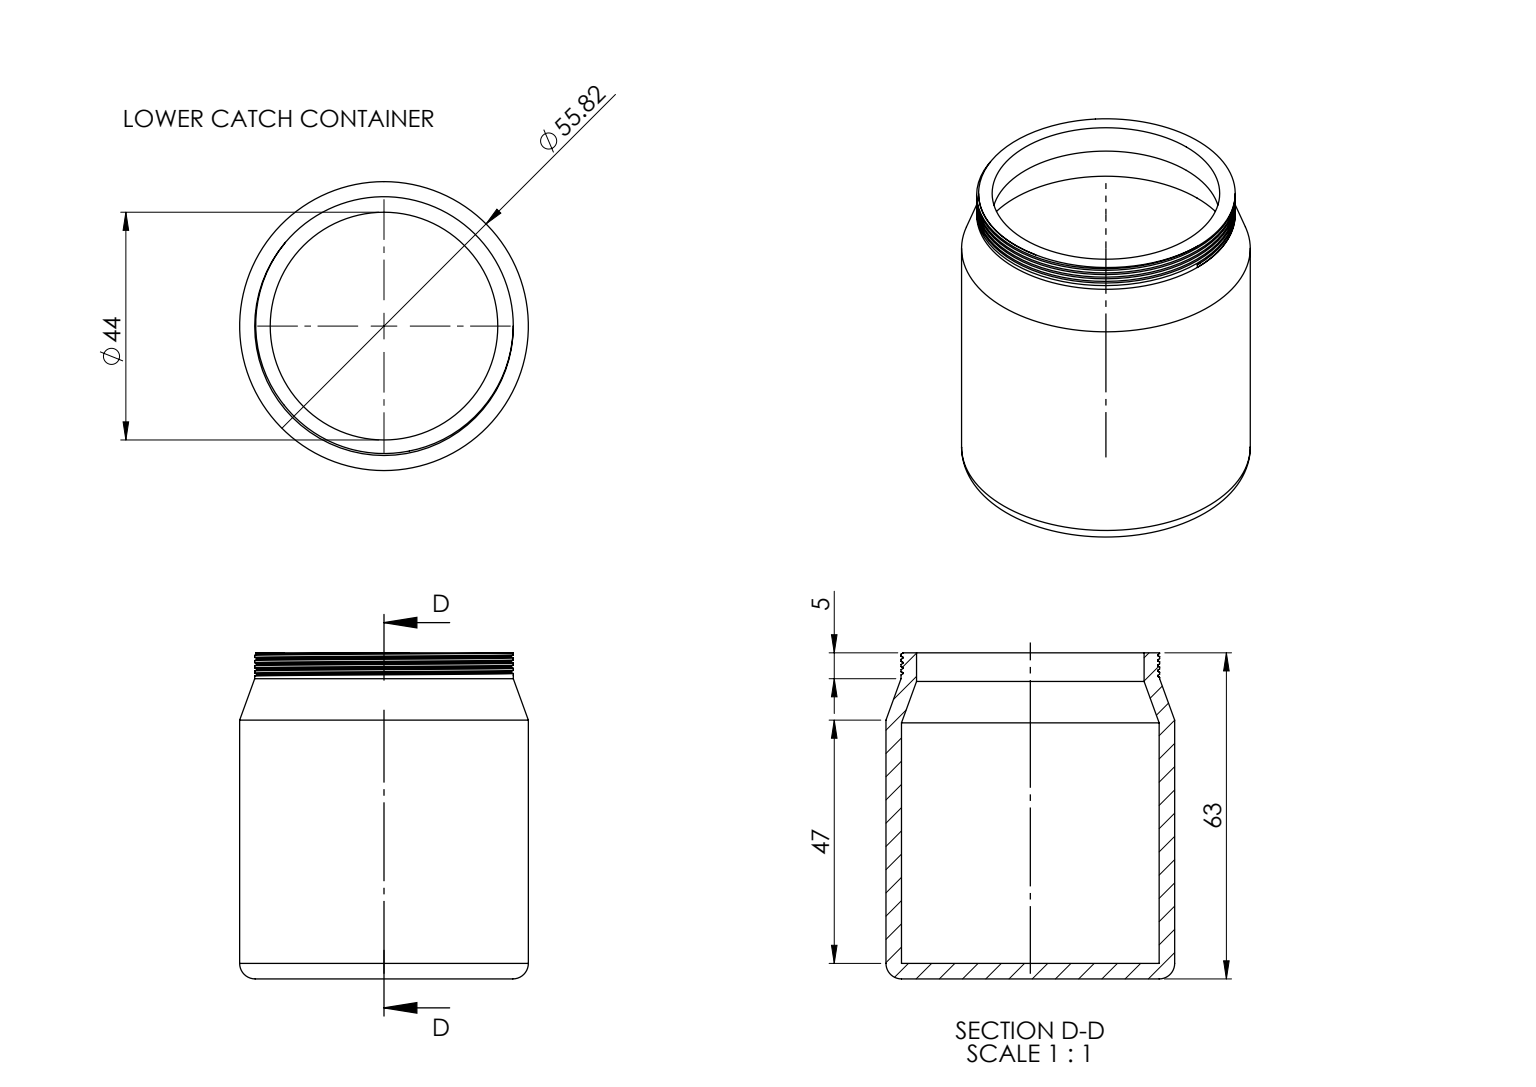
ISO-10303-21;
HEADER;
FILE_DESCRIPTION (('STEP AP214'),
    '1' );
FILE_NAME ('Lower Catch Container.step',
    '2026-10-04T07:23:31',
    ( '' ),
    ( '' ),
    'SwSTEP 2.0',
    'SolidWorks 2026',
    '' );
FILE_SCHEMA (( 'AUTOMOTIVE_DESIGN' ));
ENDSEC;

DATA;
#7=CARTESIAN_POINT ( 'NONE',  ( -10.19839929293505776, 0.5312499990440845421, -24.62111388750000174 ) ) ;
#10=CARTESIAN_POINT ( 'NONE',  ( 1.530808498934191521E-15, 3.250000000000000444, -25.00000000000000000 ) ) ;
#15=CARTESIAN_POINT ( 'NONE',  ( 24.62111388749999463, 5.156249999044083765, 10.19839929293507730 ) ) ;
#16=FACE_OUTER_BOUND ( 'NONE', #4981, .T. ) ;
#25=DIRECTION ( 'NONE',  ( 0.000000000000000000, 0.000000000000000000, -1.000000000000000000 ) ) ;
#39=VERTEX_POINT ( 'NONE', #260 ) ;
#48=TOROIDAL_SURFACE ( 'NONE', #9050, 24.91176187412963117, 3.000000000000000000 ) ;
#50=EDGE_CURVE ( 'NONE', #1424, #5838, #3619, .T. ) ;
#51=CARTESIAN_POINT ( 'NONE',  ( -10.19839929293507552, 1.081249999044084475, 24.62111388749999463 ) ) ;
#52=CARTESIAN_POINT ( 'NONE',  ( -10.19839929293505776, 1.706249999044084698, -24.62111388750000174 ) ) ;
#57=VERTEX_POINT ( 'NONE', #5944 ) ;
#59=FILL_AREA_STYLE_COLOUR ( '', #6484 ) ;
#69=VERTEX_POINT ( 'NONE', #5118 ) ;
#70=UNCERTAINTY_MEASURE_WITH_UNIT (LENGTH_MEASURE( 1.000000000000000082E-05 ), #3920, 'distance_accuracy_value', 'NONE');
#72=CARTESIAN_POINT ( 'NONE',  ( -10.19839929293507552, 0.9062499990440844311, 24.62111388749999463 ) ) ;
#79=CARTESIAN_POINT ( 'NONE',  ( 0.000000000000000000, 5.000000000000000000, 0.000000000000000000 ) ) ;
#80=CARTESIAN_POINT ( 'NONE',  ( -17.67766952966369232, 0.6250000000000000000, 17.67766952966368876 ) ) ;
#81=CARTESIAN_POINT ( 'NONE',  ( -25.00000000000000000, 3.112499998088169129, -3.061616997868383043E-15 ) ) ;
#90=FACE_OUTER_BOUND ( 'NONE', #9620, .T. ) ;
#98=CARTESIAN_POINT ( 'NONE',  ( 24.62111388750000174, 0.4562499990440845310, -10.19839929293505776 ) ) ;
#107=CARTESIAN_POINT ( 'NONE',  ( -4.522825247065398226E-15, 3.143749999044084475, 24.62111388750000174 ) ) ;
#116=CARTESIAN_POINT ( 'NONE',  ( -25.00000000000000000, 2.112499998088169129, -3.061616997868383043E-15 ) ) ;
#118=CARTESIAN_POINT ( 'NONE',  ( 17.67766952966368521, 2.875000000000000000, 17.67766952966369232 ) ) ;
#125=CARTESIAN_POINT ( 'NONE',  ( -10.19839929293507552, 5.081249999044084475, 24.62111388749999463 ) ) ;
#135=CARTESIAN_POINT ( 'NONE',  ( -25.00000000000000000, 0.4375000000000000000, -10.35533905932738108 ) ) ;
#137=EDGE_LOOP ( 'NONE', ( #3283, #4277, #3194, #1557 ) ) ;
#158=CARTESIAN_POINT ( 'NONE',  ( -24.62111388750000174, 4.831249999044084475, -10.19839929293506131 ) ) ;
#164=CARTESIAN_POINT ( 'NONE',  ( -10.19839929293505776, 0.7062499990440844755, -24.62111388750000174 ) ) ;
#166=CARTESIAN_POINT ( 'NONE',  ( -25.00000000000000000, 1.049999998088169129, -10.35533905932738108 ) ) ;
#172=CARTESIAN_POINT ( 'NONE',  ( 10.19839929293505953, 0.4062499990440845421, -24.62111388750000174 ) ) ;
#175=CARTESIAN_POINT ( 'NONE',  ( -25.00000000000001421, 3.562500000000000444, 10.35533905932737397 ) ) ;
#183=LINE ( 'NONE', #1845, #502 ) ;
#184=CARTESIAN_POINT ( 'NONE',  ( 24.62111388749999463, 4.331249999044085364, 10.19839929293507730 ) ) ;
#193=DIRECTION ( 'NONE',  ( 0.000000000000000000, 0.000000000000000000, -1.000000000000000000 ) ) ;
#195=CARTESIAN_POINT ( 'NONE',  ( -10.35533905932737575, 1.312500000000000444, -25.00000000000000000 ) ) ;
#197=CARTESIAN_POINT ( 'NONE',  ( -17.67766952966369232, 3.237499998088169573, 17.67766952966368876 ) ) ;
#204=EDGE_CURVE ( 'NONE', #10138, #4764, #1958, .T. ) ;
#218=CARTESIAN_POINT ( 'NONE',  ( 17.40975659021752975, 4.518749999044084475, -17.40975659021752975 ) ) ;
#228=CARTESIAN_POINT ( 'NONE',  ( -24.62111388750000174, 1.831249999044084475, -10.19839929293506131 ) ) ;
#237=CARTESIAN_POINT ( 'NONE',  ( -24.62111388750000174, 0.6562499990440845421, -10.19839929293506131 ) ) ;
#240=AXIS2_PLACEMENT_3D ( 'NONE', #1921, #5301, #7838 ) ;
#245=CARTESIAN_POINT ( 'NONE',  ( 17.40975659021752975, 3.518749999044084920, -17.40975659021752975 ) ) ;
#254=CARTESIAN_POINT ( 'NONE',  ( -25.00000000000000000, 1.437500000000000000, -10.35533905932738108 ) ) ;
#256=EDGE_CURVE ( 'NONE', #8849, #3847, #4015, .T. ) ;
#260=CARTESIAN_POINT ( 'NONE',  ( 1.530808498934191521E-15, 0.8624999980881691286, -25.00000000000000000 ) ) ;
#262=FACE_OUTER_BOUND ( 'NONE', #1288, .T. ) ;
#270=EDGE_LOOP ( 'NONE', ( #6260, #9302, #1877, #7015, #4822 ) ) ;
#273=CARTESIAN_POINT ( 'NONE',  ( 24.99999999999999289, 2.937500000000000000, 10.35533905932739529 ) ) ;
#274=CARTESIAN_POINT ( 'NONE',  ( 10.35533905932738286, 1.424999998088169129, 24.99999999999999645 ) ) ;
#275=CARTESIAN_POINT ( 'NONE',  ( 17.40975659021752975, 3.518749999044084920, -17.40975659021752975 ) ) ;
#282=CARTESIAN_POINT ( 'NONE',  ( 10.19839929293506486, 5.206249999044084475, 24.62111388749999819 ) ) ;
#286=ORIENTED_EDGE ( 'NONE', *, *, #9789, .F. ) ;
#289=CARTESIAN_POINT ( 'NONE',  ( -17.40975659021753330, 0.8437499990440846531, 17.40975659021752975 ) ) ;
#290=CARTESIAN_POINT ( 'NONE',  ( -10.35533905932739174, 1.299999998088169129, 24.99999999999999289 ) ) ;
#292=VERTEX_POINT ( 'NONE', #5447 ) ;
#293=CARTESIAN_POINT ( 'NONE',  ( -24.62111388750000884, 1.956249999044084475, 10.19839929293505421 ) ) ;
#296=CARTESIAN_POINT ( 'NONE',  ( -24.62111388750000174, 3.718749999044084653, -3.015216831376932151E-15 ) ) ;
#303=CARTESIAN_POINT ( 'NONE',  ( -25.00000000000001421, 4.562500000000000888, 10.35533905932737397 ) ) ;
#317=EDGE_CURVE ( 'NONE', #3676, #8924, #362, .T. ) ;
#318=EDGE_CURVE ( 'NONE', #10892, #10861, #6286, .T. ) ;
#319=EDGE_CURVE ( 'NONE', #5890, #7487, #2988, .T. ) ;
#322=CLOSED_SHELL ( 'NONE', ( #1450, #3684, #7028, #7525, #4651, #6943, #8474, #5199, #9776, #1972, #3877, #4730, #6668, #9875, #4249, #1226, #5886, #9953, #7341, #5931, #332, #8208, #7321, #2661, #1784, #4660, #4357, #1897, #2839, #1082, #8702 ) ) ;
#325=CARTESIAN_POINT ( 'NONE',  ( -10.19839929293507375, 3.081249999044084920, 24.62111388749999108 ) ) ;
#332=ADVANCED_FACE ( 'NONE', ( #499 ), #4567, .T. ) ;
#338=CARTESIAN_POINT ( 'NONE',  ( -20.27611860449447079, 4.999999999999999112, 14.06603648214180247 ) ) ;
#341=CARTESIAN_POINT ( 'NONE',  ( 3.061616997868383043E-15, 5.000000000000000000, 25.00000000000000000 ) ) ;
#344=CARTESIAN_POINT ( 'NONE',  ( -4.522825247065398226E-15, 3.968749999044084209, 24.62111388750000174 ) ) ;
#349=CARTESIAN_POINT ( 'NONE',  ( -4.522825247065398226E-15, 1.968749999044084653, 24.62111388750000174 ) ) ;
#353=LINE ( 'NONE', #3726, #6158 ) ;
#358=CARTESIAN_POINT ( 'NONE',  ( 25.00000000000000000, 2.000000000000000000, 0.000000000000000000 ) ) ;
#362=LINE ( 'NONE', #3732, #5271 ) ;
#364=VECTOR ( 'NONE', #7348, 1000.000000000000000 ) ;
#369=FACE_OUTER_BOUND ( 'NONE', #3316, .T. ) ;
#374=ORIENTED_EDGE ( 'NONE', *, *, #8125, .T. ) ;
#376=CARTESIAN_POINT ( 'NONE',  ( 17.40975659021752620, 4.268749999044084475, 17.40975659021753330 ) ) ;
#388=EDGE_CURVE ( 'NONE', #2139, #10138, #3054, .T. ) ;
#394=CARTESIAN_POINT ( 'NONE',  ( 24.62111388749999108, 2.156249999044084653, 10.19839929293507730 ) ) ;
#404=CARTESIAN_POINT ( 'NONE',  ( -17.40975659021752975, 2.593749999044084653, -17.40975659021752975 ) ) ;
#421=CARTESIAN_POINT ( 'NONE',  ( -25.00000000000001066, 0.5625000000000002220, 10.35533905932737397 ) ) ;
#434=DIRECTION ( 'NONE',  ( 0.000000000000000000, -1.000000000000000000, 0.000000000000000000 ) ) ;
#449=CARTESIAN_POINT ( 'NONE',  ( 24.62111388750000174, 4.281249999044084653, -10.19839929293505776 ) ) ;
#455=CARTESIAN_POINT ( 'NONE',  ( 1.507608415688466075E-15, 4.468749999044084653, -24.62111388750000174 ) ) ;
#466=CARTESIAN_POINT ( 'NONE',  ( -25.00000000000000000, 0.5000000000000000000, -3.061616997868383043E-15 ) ) ;
#479=MECHANICAL_DESIGN_GEOMETRIC_PRESENTATION_REPRESENTATION('',(#10362),#8224);
#480=CARTESIAN_POINT ( 'NONE',  ( -19.39162934935757931, 5.000000000000000888, 15.17115553405142947 ) ) ;
#481=DIRECTION ( 'NONE',  ( 0.000000000000000000, 0.000000000000000000, -1.000000000000000000 ) ) ;
#487=ORIENTED_EDGE ( 'NONE', *, *, #845, .F. ) ;
#498=CARTESIAN_POINT ( 'NONE',  ( 1.507608415688466075E-15, 1.468749999044084431, -24.62111388750000174 ) ) ;
#499=FACE_OUTER_BOUND ( 'NONE', #9815, .T. ) ;
#502=VECTOR ( 'NONE', #9281, 999.9999999999998863 ) ;
#503=CARTESIAN_POINT ( 'NONE',  ( 1.507608415688466075E-15, 2.468749999044085097, -24.62111388750000174 ) ) ;
#530=DIRECTION ( 'NONE',  ( -0.000000000000000000, 1.000000000000000000, -0.000000000000000000 ) ) ;
#540=STYLED_ITEM ( 'NONE', ( #5737 ), #3340 ) ;
#547=CARTESIAN_POINT ( 'NONE',  ( 24.62111388750000174, 1.281249999044084653, -10.19839929293505776 ) ) ;
#552=CARTESIAN_POINT ( 'NONE',  ( -25.00000000000001421, 3.174999998088169129, 10.35533905932737397 ) ) ;
#560=DIRECTION ( 'NONE',  ( 0.000000000000000000, 0.000000000000000000, -1.000000000000000000 ) ) ;
#563=ORIENTED_EDGE ( 'NONE', *, *, #319, .T. ) ;
#568=CARTESIAN_POINT ( 'NONE',  ( 25.00000000000000000, 4.000000000000000000, 0.000000000000000000 ) ) ;
#589=CIRCLE ( 'NONE', #3780, 22.00000000000000355 ) ;
#596=ORIENTED_EDGE ( 'NONE', *, *, #10438, .T. ) ;
#609=CARTESIAN_POINT ( 'NONE',  ( -25.00000000000000000, 5.112499998088170017, -3.061616997868383043E-15 ) ) ;
#627=CYLINDRICAL_SURFACE ( 'NONE', #9189, 25.00000000000000000 ) ;
#629=CARTESIAN_POINT ( 'NONE',  ( 24.62111388749999463, 2.156249999044085097, 10.19839929293507730 ) ) ;
#630=CARTESIAN_POINT ( 'NONE',  ( 1.530808498934191521E-15, 3.250000000000000444, -25.00000000000000000 ) ) ;
#657=CARTESIAN_POINT ( 'NONE',  ( -17.67766952966369232, 1.625000000000000222, 17.67766952966368876 ) ) ;
#662=CARTESIAN_POINT ( 'NONE',  ( -24.62111388750000884, 0.9562499990440846975, 10.19839929293505421 ) ) ;
#676=ORIENTED_EDGE ( 'NONE', *, *, #388, .T. ) ;
#686=CARTESIAN_POINT ( 'NONE',  ( 24.62111388750000174, 3.218749999044084653, 0.000000000000000000 ) ) ;
#704=CARTESIAN_POINT ( 'NONE',  ( -17.40975659021752975, 0.7687499990440845865, -17.40975659021752975 ) ) ;
#708=PLANE ( 'NONE',  #6776 ) ;
#718=CARTESIAN_POINT ( 'NONE',  ( -10.35533905932737575, 3.924999998088169129, -25.00000000000000000 ) ) ;
#733=PRODUCT_DEFINITION_CONTEXT ( 'detailed design', #2156, 'design' ) ;
#738=EDGE_CURVE ( 'NONE', #69, #8014, #353, .T. ) ;
#739=AXIS2_PLACEMENT_3D ( 'NONE', #4438, #9619, #4506 ) ;
#743=CARTESIAN_POINT ( 'NONE',  ( -24.62111388750000884, 0.7812499990440845421, 10.19839929293505421 ) ) ;
#747=ORIENTED_EDGE ( 'NONE', *, *, #1322, .F. ) ;
#763=DIRECTION ( 'NONE',  ( 0.000000000000000000, -1.000000000000000000, 0.000000000000000000 ) ) ;
#764=CARTESIAN_POINT ( 'NONE',  ( 1.530808498934191521E-15, 4.862499998088169129, -25.00000000000000000 ) ) ;
#765=LINE ( 'NONE', #10659, #3839 ) ;
#779=CARTESIAN_POINT ( 'NONE',  ( -17.40975659021752975, 0.7687499990440845865, -17.40975659021752975 ) ) ;
#800=CARTESIAN_POINT ( 'NONE',  ( 0.000000000000000000, -0.5289809421253948152, -22.00000000000000355 ) ) ;
#804=CARTESIAN_POINT ( 'NONE',  ( 1.507608415688466075E-15, 2.468749999044085097, -24.62111388750000174 ) ) ;
#825=CYLINDRICAL_SURFACE ( 'NONE', #10417, 25.00000000000000000 ) ;
#830=CARTESIAN_POINT ( 'NONE',  ( 1.507608415688466075E-15, 3.643749999044084920, -24.62111388750000174 ) ) ;
#834=EDGE_LOOP ( 'NONE', ( #2403, #1954, #8733, #10680 ) ) ;
#844=CARTESIAN_POINT ( 'NONE',  ( 1.507608415688466075E-15, 0.4687499990440845421, -24.62111388750000174 ) ) ;
#845=EDGE_CURVE ( 'NONE', #8849, #1367, #2420, .T. ) ;
#850=CARTESIAN_POINT ( 'NONE',  ( 0.000000000000000000, -55.00000000000000000, 0.000000000000000000 ) ) ;
#853=CARTESIAN_POINT ( 'NONE',  ( -10.19839929293507552, 3.906249999044085097, 24.62111388749999463 ) ) ;
#866=CYLINDRICAL_SURFACE ( 'NONE', #8002, 22.00000000000000355 ) ;
#886=CARTESIAN_POINT ( 'NONE',  ( 10.19839929293505953, 0.5812499990440845865, -24.62111388750000174 ) ) ;
#887=CARTESIAN_POINT ( 'NONE',  ( -17.40975659021753330, 2.018749999044084475, 17.40975659021752975 ) ) ;
#889=CARTESIAN_POINT ( 'NONE',  ( -25.00000000000000000, 1.112499998088169351, -3.061616997868383043E-15 ) ) ;
#893=FILL_AREA_STYLE ('',( #59 ) ) ;
#904=CARTESIAN_POINT ( 'NONE',  ( 24.62111388749999463, 2.331249999044084031, 10.19839929293507730 ) ) ;
#912=CARTESIAN_POINT ( 'NONE',  ( 25.00000000000000000, 4.674999998088169129, -10.35533905932737753 ) ) ;
#913=CARTESIAN_POINT ( 'NONE',  ( 1.530808498934191521E-15, 2.862499998088169573, -25.00000000000000000 ) ) ;
#914=ORIENTED_EDGE ( 'NONE', *, *, #10318, .T. ) ;
#924=CARTESIAN_POINT ( 'NONE',  ( 10.35533905932740240, 1.812500000000000222, 24.99999999999998224 ) ) ;
#929=CARTESIAN_POINT ( 'NONE',  ( 11.57348645726024117, 5.000000000000000888, 21.83446729476942139 ) ) ;
#950=CARTESIAN_POINT ( 'NONE',  ( 24.62111388750000174, 1.393749999044084475, 0.000000000000000000 ) ) ;
#951=CARTESIAN_POINT ( 'NONE',  ( 10.19839929293505953, 1.581249999044084475, -24.62111388750000174 ) ) ;
#960=CARTESIAN_POINT ( 'NONE',  ( -25.00000000000000000, 2.049999998088169129, -10.35533905932738108 ) ) ;
#962=CARTESIAN_POINT ( 'NONE',  ( 17.67766952966369232, 4.125000000000000000, -17.67766952966369232 ) ) ;
#969=CARTESIAN_POINT ( 'NONE',  ( 10.19839929293505953, 4.581249999044085364, -24.62111388750000174 ) ) ;
#985=DIRECTION ( 'NONE',  ( 0.000000000000000000, 0.000000000000000000, -1.000000000000000000 ) ) ;
#995=CARTESIAN_POINT ( 'NONE',  ( -10.19839929293507375, 4.081249999044084475, 24.62111388749999108 ) ) ;
#1003=CARTESIAN_POINT ( 'NONE',  ( -17.40975659021752975, 1.768749999044084475, -17.40975659021752975 ) ) ;
#1007=ORIENTED_EDGE ( 'NONE', *, *, #4743, .T. ) ;
#1015=CARTESIAN_POINT ( 'NONE',  ( 24.99999999999999289, 3.937500000000000000, 10.35533905932739529 ) ) ;
#1021=CARTESIAN_POINT ( 'NONE',  ( -24.62111388750000174, 3.893749999044084475, -3.015216831376932151E-15 ) ) ;
#1027=DIRECTION ( 'NONE',  ( 0.000000000000000000, -1.000000000000000000, 0.000000000000000000 ) ) ;
#1030=CARTESIAN_POINT ( 'NONE',  ( 17.40975659021752975, 4.343749999044084653, -17.40975659021752975 ) ) ;
#1051=CARTESIAN_POINT ( 'NONE',  ( -4.522825247065398226E-15, 1.143749999044084475, 24.62111388750000174 ) ) ;
#1059=CARTESIAN_POINT ( 'NONE',  ( -10.19839929293505776, 1.706249999044084698, -24.62111388750000174 ) ) ;
#1060=CARTESIAN_POINT ( 'NONE',  ( -10.19839929293507552, 4.081249999044084475, 24.62111388749999463 ) ) ;
#1062=LINE ( 'NONE', #7619, #7030 ) ;
#1070=CARTESIAN_POINT ( 'NONE',  ( 10.35533905932737930, 3.187500000000000000, -25.00000000000000000 ) ) ;
#1078=CARTESIAN_POINT ( 'NONE',  ( -17.40975659021753330, 5.018749999044084475, 17.40975659021752975 ) ) ;
#1082=ADVANCED_FACE ( 'NONE', ( #10116 ), #9716, .T. ) ;
#1083=VECTOR ( 'NONE', #8766, 1000.000000000000000 ) ;
#1089=CARTESIAN_POINT ( 'NONE',  ( -10.19839929293507552, 4.906249999044083765, 24.62111388749999463 ) ) ;
#1090=CARTESIAN_POINT ( 'NONE',  ( 3.050810944027392283E-15, -8.528980942125404141, 24.91176187412963117 ) ) ;
#1094=AXIS2_PLACEMENT_3D ( 'NONE', #5441, #5400, #9532 ) ;
#1096=EDGE_CURVE ( 'NONE', #8849, #8924, #1941, .T. ) ;
#1097=DIRECTION ( 'NONE',  ( 0.000000000000000000, -1.000000000000000000, 0.000000000000000000 ) ) ;
#1105=ORIENTED_EDGE ( 'NONE', *, *, #4602, .T. ) ;
#1108=CARTESIAN_POINT ( 'NONE',  ( 25.00000000000000000, 1.674999998088169351, -10.35533905932737753 ) ) ;
#1110=CARTESIAN_POINT ( 'NONE',  ( -17.40975659021752975, 3.768749999044084475, -17.40975659021752975 ) ) ;
#1120=CARTESIAN_POINT ( 'NONE',  ( -10.35533905932737575, 0.9249999980881692396, -25.00000000000000000 ) ) ;
#1124=DIRECTION ( 'NONE',  ( 0.000000000000000000, 0.000000000000000000, -1.000000000000000000 ) ) ;
#1126=CARTESIAN_POINT ( 'NONE',  ( -24.62111388750000174, 0.7187499990440845421, -3.015216831376932151E-15 ) ) ;
#1138=CARTESIAN_POINT ( 'NONE',  ( -24.62111388750000884, 1.781249999044084431, 10.19839929293505421 ) ) ;
#1148=CARTESIAN_POINT ( 'NONE',  ( 1.530808498934191521E-15, 2.250000000000000444, -25.00000000000000000 ) ) ;
#1149=CARTESIAN_POINT ( 'NONE',  ( -4.592425496802574367E-15, 4.750000000000000000, 25.00000000000000000 ) ) ;
#1151=CARTESIAN_POINT ( 'NONE',  ( -17.67766952966368876, 2.375000000000000000, -17.67766952966369232 ) ) ;
#1168=CARTESIAN_POINT ( 'NONE',  ( 25.00000000000000000, 1.612499998088169351, 0.000000000000000000 ) ) ;
#1169=CARTESIAN_POINT ( 'NONE',  ( 24.62111388750000174, 1.456249999044084920, -10.19839929293505776 ) ) ;
#1172=DIRECTION ( 'NONE',  ( 0.000000000000000000, -1.000000000000000000, 0.000000000000000000 ) ) ;
#1174=CARTESIAN_POINT ( 'NONE',  ( -24.62111388750000174, 4.893749999044084475, -3.015216831376932151E-15 ) ) ;
#1176=CARTESIAN_POINT ( 'NONE',  ( -20.77469822633729279, 4.999999999999997335, -13.92348360573865840 ) ) ;
#1181=CARTESIAN_POINT ( 'NONE',  ( 10.19839929293505953, 4.406249999044084653, -24.62111388750000174 ) ) ;
#1186=CARTESIAN_POINT ( 'NONE',  ( 24.62111388750000174, 4.281249999044084653, -10.19839929293505776 ) ) ;
#1200=CARTESIAN_POINT ( 'NONE',  ( 3.050810944027392283E-15, -55.00000000000000000, 24.91176187412963117 ) ) ;
#1201=CARTESIAN_POINT ( 'NONE',  ( -10.35533905932737575, 3.924999998088168685, -25.00000000000000000 ) ) ;
#1214=CARTESIAN_POINT ( 'NONE',  ( -10.19839929293505776, 2.706249999044084475, -24.62111388750000174 ) ) ;
#1222=EDGE_LOOP ( 'NONE', ( #9049, #9429 ) ) ;
#1224=CARTESIAN_POINT ( 'NONE',  ( -24.71676035596633270, 5.000000000000000000, 2.273299333383253185 ) ) ;
#1226=ADVANCED_FACE ( 'NONE', ( #10148 ), #2458, .T. ) ;
#1230=CARTESIAN_POINT ( 'NONE',  ( -10.19839929293505776, 4.531249999044084653, -24.62111388750000174 ) ) ;
#1233=ORIENTED_EDGE ( 'NONE', *, *, #8133, .T. ) ;
#1235=CARTESIAN_POINT ( 'NONE',  ( -17.40975659021753330, 3.843749999044085097, 17.40975659021752975 ) ) ;
#1243=TOROIDAL_SURFACE ( 'NONE', #1944, 24.91176187412963117, 3.000000000000000000 ) ;
#1244=EDGE_LOOP ( 'NONE', ( #5826, #1663, #6426, #7459 ) ) ;
#1252=LINE ( 'NONE', #1354, #7425 ) ;
#1262=FACE_OUTER_BOUND ( 'NONE', #7179, .T. ) ;
#1273=CARTESIAN_POINT ( 'NONE',  ( 0.000000000000000000, -58.00000000000000000, 27.91176187412963117 ) ) ;
#1275=CARTESIAN_POINT ( 'NONE',  ( -19.39162934935757931, 5.000000000000000888, 15.17115553405142947 ) ) ;
#1282=CARTESIAN_POINT ( 'NONE',  ( 17.40975659021752620, 3.093749999044084653, 17.40975659021753330 ) ) ;
#1288=EDGE_LOOP ( 'NONE', ( #4925, #3557, #374, #9513 ) ) ;
#1289=AXIS2_PLACEMENT_3D ( 'NONE', #7063, #7010, #10421 ) ;
#1291=CARTESIAN_POINT ( 'NONE',  ( 17.40975659021752620, 3.093749999044084653, 17.40975659021753330 ) ) ;
#1295=DIRECTION ( 'NONE',  ( 0.000000000000000000, -1.000000000000000000, 0.000000000000000000 ) ) ;
#1306=CARTESIAN_POINT ( 'NONE',  ( -17.67766952966369232, 4.237499998088169129, 17.67766952966368876 ) ) ;
#1322=EDGE_CURVE ( 'NONE', #6596, #4397, #183, .T. ) ;
#1323=CARTESIAN_POINT ( 'NONE',  ( 0.000000000000000000, -55.00000000000000000, -24.91176187412963117 ) ) ;
#1328=CARTESIAN_POINT ( 'NONE',  ( 1.530808498934191521E-15, 2.862499998088169573, -25.00000000000000000 ) ) ;
#1329=CARTESIAN_POINT ( 'NONE',  ( 24.62111388750000174, 1.218749999044084431, 0.000000000000000000 ) ) ;
#1330=CARTESIAN_POINT ( 'NONE',  ( 17.67766952966369232, 0.1249999999999999722, -17.67766952966369232 ) ) ;
#1338=CARTESIAN_POINT ( 'NONE',  ( -17.40975659021752975, 4.593749999044084653, -17.40975659021752975 ) ) ;
#1349=CARTESIAN_POINT ( 'NONE',  ( -17.67766952966368876, 0.3750000000000000000, -17.67766952966369232 ) ) ;
#1354=CARTESIAN_POINT ( 'NONE',  ( 24.81055694375000087, 0.5031249985661269131, 0.000000000000000000 ) ) ;
#1355=CARTESIAN_POINT ( 'NONE',  ( 17.40975659021752975, 0.3437499990440845421, -17.40975659021752975 ) ) ;
#1359=ORIENTED_EDGE ( 'NONE', *, *, #2795, .T. ) ;
#1361=CARTESIAN_POINT ( 'NONE',  ( 0.000000000000000000, 0.000000000000000000, -25.00000000000000000 ) ) ;
#1367=VERTEX_POINT ( 'NONE', #1726 ) ;
#1369=CARTESIAN_POINT ( 'NONE',  ( -19.05903902044739695, 4.999999999999999112, -16.17878337876688022 ) ) ;
#1375=CARTESIAN_POINT ( 'NONE',  ( 10.19839929293505953, 2.406249999044085541, -24.62111388750000174 ) ) ;
#1381=CARTESIAN_POINT ( 'NONE',  ( -24.62111388750000174, 0.8312499990440843645, -10.19839929293506131 ) ) ;
#1393=ORIENTED_EDGE ( 'NONE', *, *, #3624, .T. ) ;
#1399=CARTESIAN_POINT ( 'NONE',  ( 17.67766952966369232, 1.737499998088169351, -17.67766952966369232 ) ) ;
#1406=AXIS2_PLACEMENT_3D ( 'NONE', #1323, #7180, #10444 ) ;
#1415=CARTESIAN_POINT ( 'NONE',  ( -4.592425496802574367E-15, 0.7500000000000000000, 25.00000000000000000 ) ) ;
#1420=( NAMED_UNIT ( * ) SI_UNIT ( $, .STERADIAN. ) SOLID_ANGLE_UNIT ( ) );
#1423=CARTESIAN_POINT ( 'NONE',  ( 24.99999999999999289, 2.549999998088169129, 10.35533905932739529 ) ) ;
#1424=VERTEX_POINT ( 'NONE', #2760 ) ;
#1430=CARTESIAN_POINT ( 'NONE',  ( 1.530808498934191521E-15, 4.862499998088169129, -25.00000000000000000 ) ) ;
#1450=ADVANCED_FACE ( 'NONE', ( #6159 ), #10559, .F. ) ;
#1454=CARTESIAN_POINT ( 'NONE',  ( 3.061616997868383043E-15, 0.000000000000000000, 25.00000000000000000 ) ) ;
#1462=CARTESIAN_POINT ( 'NONE',  ( -10.19839929293505776, 0.5312499990440845421, -24.62111388750000174 ) ) ;
#1463=CARTESIAN_POINT ( 'NONE',  ( -25.00000000000001066, 3.562500000000000000, 10.35533905932737397 ) ) ;
#1469=ORIENTED_EDGE ( 'NONE', *, *, #10521, .T. ) ;
#1473=VECTOR ( 'NONE', #5246, 1000.000000000000000 ) ;
#1494=CARTESIAN_POINT ( 'NONE',  ( -25.00000000000000000, 3.049999998088169129, -10.35533905932738108 ) ) ;
#1495=CARTESIAN_POINT ( 'NONE',  ( 24.62111388750000174, 5.218749999044084653, 0.000000000000000000 ) ) ;
#1507=CARTESIAN_POINT ( 'NONE',  ( 0.3808229674253814645, 5.000000000000004441, 24.72275166764144316 ) ) ;
#1509=CARTESIAN_POINT ( 'NONE',  ( 10.19839929293505953, 0.4062499990440845421, -24.62111388750000174 ) ) ;
#1520=CARTESIAN_POINT ( 'NONE',  ( 10.35533905932737930, 1.187500000000000000, -25.00000000000000000 ) ) ;
#1524=ORIENTED_EDGE ( 'NONE', *, *, #3129, .T. ) ;
#1526=SURFACE_SIDE_STYLE ('',( #9925 ) ) ;
#1528=CARTESIAN_POINT ( 'NONE',  ( 10.19839929293505953, 0.5812499990440844755, -24.62111388750000174 ) ) ;
#1535=CARTESIAN_POINT ( 'NONE',  ( -25.00000000000001066, 1.562500000000000000, 10.35533905932737397 ) ) ;
#1542=CARTESIAN_POINT ( 'NONE',  ( 10.35533905932737930, 3.799999998088170017, -25.00000000000000000 ) ) ;
#1543=CARTESIAN_POINT ( 'NONE',  ( 0.000000000000000000, 0.000000000000000000, 0.000000000000000000 ) ) ;
#1557=ORIENTED_EDGE ( 'NONE', *, *, #2141, .T. ) ;
#1561=CARTESIAN_POINT ( 'NONE',  ( -10.65103055884460836, 4.999999999999998224, 22.31395431344387603 ) ) ;
#1564=CARTESIAN_POINT ( 'NONE',  ( -4.522825247065398226E-15, 3.968749999044084209, 24.62111388750000174 ) ) ;
#1572=CARTESIAN_POINT ( 'NONE',  ( 0.000000000000000000, -8.000000000000000000, 0.000000000000000000 ) ) ;
#1574=CARTESIAN_POINT ( 'NONE',  ( 10.29762009200904949, 5.000000000000000000, 22.44659794629365024 ) ) ;
#1579=CARTESIAN_POINT ( 'NONE',  ( 0.000000000000000000, 5.000000000000000000, 0.000000000000000000 ) ) ;
#1583=ORIENTED_EDGE ( 'NONE', *, *, #3129, .F. ) ;
#1585=CARTESIAN_POINT ( 'NONE',  ( 17.67766952966368521, 3.487499998088169129, 17.67766952966369232 ) ) ;
#1597=CARTESIAN_POINT ( 'NONE',  ( 17.67766952966368521, 5.487499998088169129, 17.67766952966369232 ) ) ;
#1612=ORIENTED_EDGE ( 'NONE', *, *, #9694, .F. ) ;
#1620=CARTESIAN_POINT ( 'NONE',  ( -25.00000000000000000, 2.049999998088169129, -10.35533905932738108 ) ) ;
#1624=CARTESIAN_POINT ( 'NONE',  ( 24.62111388749999463, 1.156249999044084431, 10.19839929293507730 ) ) ;
#1628=ORIENTED_EDGE ( 'NONE', *, *, #9519, .T. ) ;
#1632=ORIENTED_EDGE ( 'NONE', *, *, #1723, .T. ) ;
#1634=AXIS2_PLACEMENT_3D ( 'NONE', #5503, #2126, #5669 ) ;
#1639=CARTESIAN_POINT ( 'NONE',  ( 24.99258498528540429, 4.999999999999999112, 0.7093093681917175264 ) ) ;
#1642=VERTEX_POINT ( 'NONE', #8656 ) ;
#1646=CARTESIAN_POINT ( 'NONE',  ( -10.35533905932735621, 4.687500000000000888, 25.00000000000003197 ) ) ;
#1652=CARTESIAN_POINT ( 'NONE',  ( -10.35533905932737220, 1.687500000000000222, 25.00000000000001421 ) ) ;
#1655=ORIENTED_EDGE ( 'NONE', *, *, #738, .F. ) ;
#1659=CARTESIAN_POINT ( 'NONE',  ( -10.19839929293505776, 4.706249999044084475, -24.62111388750000174 ) ) ;
#1663=ORIENTED_EDGE ( 'NONE', *, *, #8734, .F. ) ;
#1683=CARTESIAN_POINT ( 'NONE',  ( -24.62111388750000174, 3.718749999044084653, -3.015216831376932151E-15 ) ) ;
#1688=ORIENTED_EDGE ( 'NONE', *, *, #5712, .F. ) ;
#1702=DIRECTION ( 'NONE',  ( -0.000000000000000000, 1.000000000000000000, -0.000000000000000000 ) ) ;
#1706=CARTESIAN_POINT ( 'NONE',  ( -24.62111388750000884, 1.956249999044084475, 10.19839929293505421 ) ) ;
#1711=DIRECTION ( 'NONE',  ( 0.000000000000000000, 0.000000000000000000, -1.000000000000000000 ) ) ;
#1716=CARTESIAN_POINT ( 'NONE',  ( 25.00000000000000000, 1.674999998088169351, -10.35533905932737753 ) ) ;
#1723=EDGE_CURVE ( 'NONE', #5890, #9754, #7660, .T. ) ;
#1726=CARTESIAN_POINT ( 'NONE',  ( 3.418204983771598122E-15, -55.00000000000000000, -27.91176187412963117 ) ) ;
#1727=CARTESIAN_POINT ( 'NONE',  ( 17.40975659021752620, 3.268749999044084475, 17.40975659021753330 ) ) ;
#1736=CARTESIAN_POINT ( 'NONE',  ( 10.35533905932738286, 1.812500000000000222, 24.99999999999999645 ) ) ;
#1746=LINE ( 'NONE', #7490, #1473 ) ;
#1751=CARTESIAN_POINT ( 'NONE',  ( 18.79565575497285224, 5.000000000000000000, 16.19935794129608908 ) ) ;
#1772=CARTESIAN_POINT ( 'NONE',  ( 17.40975659021752975, 4.518749999044084475, -17.40975659021752975 ) ) ;
#1778=CARTESIAN_POINT ( 'NONE',  ( -25.00000000000000000, 1.049999998088169129, -10.35533905932738108 ) ) ;
#1784=ADVANCED_FACE ( 'NONE', ( #369 ), #3334, .F. ) ;
#1786=CARTESIAN_POINT ( 'NONE',  ( 24.62111388750000174, 3.393749999044084475, 0.000000000000000000 ) ) ;
#1794=CARTESIAN_POINT ( 'NONE',  ( 4.895565917430008795, 5.000000000000001776, 24.12949820052922334 ) ) ;
#1795=CARTESIAN_POINT ( 'NONE',  ( -10.35533905932737575, 2.312500000000000888, -25.00000000000000000 ) ) ;
#1796=CARTESIAN_POINT ( 'NONE',  ( 1.507608415688466075E-15, 4.468749999044084653, -24.62111388750000174 ) ) ;
#1805=CARTESIAN_POINT ( 'NONE',  ( -25.00000000000001066, 4.174999998088169129, 10.35533905932737397 ) ) ;
#1817=VECTOR ( 'NONE', #6504, 1000.000000000000114 ) ;
#1821=CARTESIAN_POINT ( 'NONE',  ( 10.19839929293506486, 1.206249999044084698, 24.62111388749999819 ) ) ;
#1822=( BOUNDED_CURVE ( )  B_SPLINE_CURVE ( 2, ( #10813, #10143, #4235, #5074, #9193 ),
 .UNSPECIFIED., .F., .F. ) 
 B_SPLINE_CURVE_WITH_KNOTS ( ( 3, 2, 3 ),
 ( 0.9500000000000000666, 0.9750000000000000888, 1.000000000000000000 ),
 .UNSPECIFIED. ) 
 CURVE ( )  GEOMETRIC_REPRESENTATION_ITEM ( )  RATIONAL_B_SPLINE_CURVE ( ( 0.9999999999999996669, 0.9238795325112870716, 1.000000000000000000, 0.9238795325112867385, 1.000000000000000000 ) ) 
 REPRESENTATION_ITEM ( '' )  );
#1832=CARTESIAN_POINT ( 'NONE',  ( -17.40975659021752975, 3.768749999044084475, -17.40975659021752975 ) ) ;
#1842=CARTESIAN_POINT ( 'NONE',  ( 10.35533905932738286, 3.812500000000000000, 24.99999999999999645 ) ) ;
#1845=CARTESIAN_POINT ( 'NONE',  ( 0.000000000000000000, 0.000000000000000000, -25.00000000000000000 ) ) ;
#1846=CARTESIAN_POINT ( 'NONE',  ( 24.62111388749999463, 3.331249999044084920, 10.19839929293507730 ) ) ;
#1863=ORIENTED_EDGE ( 'NONE', *, *, #2250, .F. ) ;
#1871=ORIENTED_EDGE ( 'NONE', *, *, #5325, .F. ) ;
#1876=CARTESIAN_POINT ( 'NONE',  ( 17.40975659021752975, 1.518749999044084698, -17.40975659021752975 ) ) ;
#1877=ORIENTED_EDGE ( 'NONE', *, *, #8898, .F. ) ;
#1884=CARTESIAN_POINT ( 'NONE',  ( -4.522825247065398226E-15, 4.143749999044083587, 24.62111388750000174 ) ) ;
#1890=( LENGTH_UNIT ( ) NAMED_UNIT ( * ) SI_UNIT ( .MILLI., .METRE. ) );
#1891=PLANE ( 'NONE',  #10641 ) ;
#1892=CARTESIAN_POINT ( 'NONE',  ( -17.40975659021752975, 0.5937499990440846531, -17.40975659021752975 ) ) ;
#1894=CARTESIAN_POINT ( 'NONE',  ( -17.67766952966369232, 2.625000000000000000, 17.67766952966368876 ) ) ;
#1897=ADVANCED_FACE ( 'NONE', ( #4692 ), #10067, .T. ) ;
#1900=CARTESIAN_POINT ( 'NONE',  ( -24.62111388750000884, 3.956249999044084920, 10.19839929293505421 ) ) ;
#1904=CARTESIAN_POINT ( 'NONE',  ( 0.000000000000000000, 0.000000000000000000, 0.000000000000000000 ) ) ;
#1907=FACE_OUTER_BOUND ( 'NONE', #6597, .T. ) ;
#1908=CARTESIAN_POINT ( 'NONE',  ( 25.00000000000000000, 5.000000000000000000, 0.000000000000000000 ) ) ;
#1909=CARTESIAN_POINT ( 'NONE',  ( -4.592425496802574367E-15, 3.362499998088169129, 25.00000000000000000 ) ) ;
#1910=ORIENTED_EDGE ( 'NONE', *, *, #6520, .F. ) ;
#1921=CARTESIAN_POINT ( 'NONE',  ( 0.000000000000000000, -55.00000000000000000, 0.000000000000000000 ) ) ;
#1932=CARTESIAN_POINT ( 'NONE',  ( 24.62111388750000174, 4.456249999044084475, -10.19839929293505776 ) ) ;
#1941=LINE ( 'NONE', #1273, #8795 ) ;
#1944=AXIS2_PLACEMENT_3D ( 'NONE', #4338, #7926, #5175 ) ;
#1946=ORIENTED_EDGE ( 'NONE', *, *, #2141, .F. ) ;
#1951=CARTESIAN_POINT ( 'NONE',  ( -10.35533905932737575, 0.9249999980881692396, -25.00000000000000000 ) ) ;
#1954=ORIENTED_EDGE ( 'NONE', *, *, #5712, .T. ) ;
#1957=CIRCLE ( 'NONE', #6896, 24.91176187412963117 ) ;
#1958=( BOUNDED_CURVE ( )  B_SPLINE_CURVE ( 2, ( #3890, #10574, #1349, #10627, #466, #421, #3042, #9793, #6389 ),
 .UNSPECIFIED., .F., .F. ) 
 B_SPLINE_CURVE_WITH_KNOTS ( ( 3, 2, 2, 2, 3 ),
 ( 0.05000000000000000278, 0.07500000000000001110, 0.1000000000000000194, 0.1250000000000000278, 0.1500000000000000222 ),
 .UNSPECIFIED. ) 
 CURVE ( )  GEOMETRIC_REPRESENTATION_ITEM ( )  RATIONAL_B_SPLINE_CURVE ( ( 1.000000000000000000, 0.9238795325112867385, 1.000000000000000000, 0.9238795325112867385, 1.000000000000000000, 0.9238795325112867385, 1.000000000000000000, 0.9238795325112866275, 1.000000000000000000 ) ) 
 REPRESENTATION_ITEM ( '' )  );
#1961=CARTESIAN_POINT ( 'NONE',  ( 24.62111388750000174, 2.218749999044084653, 0.000000000000000000 ) ) ;
#1971=CYLINDRICAL_SURFACE ( 'NONE', #1094, 25.00000000000000000 ) ;
#1972=ADVANCED_FACE ( 'NONE', ( #8581 ), #1971, .T. ) ;
#1973=CARTESIAN_POINT ( 'NONE',  ( -17.67766952966369232, 1.625000000000000222, 17.67766952966368876 ) ) ;
#1974=CARTESIAN_POINT ( 'NONE',  ( -10.35533905932739174, 3.299999998088169129, 24.99999999999999289 ) ) ;
#1992=CARTESIAN_POINT ( 'NONE',  ( 10.19839929293505953, 2.581249999044084920, -24.62111388750000174 ) ) ;
#1993=ORIENTED_EDGE ( 'NONE', *, *, #4111, .T. ) ;
#2000=ORIENTED_EDGE ( 'NONE', *, *, #4111, .F. ) ;
#2002=VECTOR ( 'NONE', #6089, 1000.000000000000000 ) ;
#2004=CARTESIAN_POINT ( 'NONE',  ( -24.13837508890848227, 4.999999999999997335, -6.164697453113522130 ) ) ;
#2010=CARTESIAN_POINT ( 'NONE',  ( -17.40975659021752975, 1.593749999044084431, -17.40975659021752975 ) ) ;
#2014=AXIS2_PLACEMENT_3D ( 'NONE', #4180, #7777, #985 ) ;
#2019=CARTESIAN_POINT ( 'NONE',  ( -17.40975659021753330, 4.843749999044083765, 17.40975659021752975 ) ) ;
#2022=AXIS2_PLACEMENT_3D ( 'NONE', #3911, #530, #4800 ) ;
#2035=CARTESIAN_POINT ( 'NONE',  ( 24.62111388750000174, 0.2187499990440845699, 0.000000000000000000 ) ) ;
#2038=VERTEX_POINT ( 'NONE', #7823 ) ;
#2041=CARTESIAN_POINT ( 'NONE',  ( 24.62111388749999108, 3.331249999044084920, 10.19839929293507730 ) ) ;
#2054=CARTESIAN_POINT ( 'NONE',  ( -24.62111388750000174, 4.718749999044084653, -3.015216831376932151E-15 ) ) ;
#2057=CARTESIAN_POINT ( 'NONE',  ( -24.62111388750000884, 2.781249999044085541, 10.19839929293505421 ) ) ;
#2093=CARTESIAN_POINT ( 'NONE',  ( -22.78663523973255067, 5.000000000000000888, -10.19028184728269437 ) ) ;
#2097=DIRECTION ( 'NONE',  ( 0.000000000000000000, -0.000000000000000000, -1.000000000000000000 ) ) ;
#2099=CARTESIAN_POINT ( 'NONE',  ( -24.62111388750000174, 3.718749999044084653, -3.015216831376932151E-15 ) ) ;
#2100=CARTESIAN_POINT ( 'NONE',  ( 10.35533905932734733, 4.187500000000000888, -25.00000000000004263 ) ) ;
#2105=CARTESIAN_POINT ( 'NONE',  ( -24.62111388750000884, 3.781249999044084653, 10.19839929293505421 ) ) ;
#2115=CARTESIAN_POINT ( 'NONE',  ( -25.00000000000000000, 2.437500000000000444, -10.35533905932738108 ) ) ;
#2118=CARTESIAN_POINT ( 'NONE',  ( 0.000000000000000000, -1.026060429977008193, -22.18092213764227694 ) ) ;
#2126=DIRECTION ( 'NONE',  ( 0.000000000000000000, -1.000000000000000000, 0.000000000000000000 ) ) ;
#2134=DIRECTION ( 'NONE',  ( 0.000000000000000000, -1.000000000000000000, 0.000000000000000000 ) ) ;
#2136=LINE ( 'NONE', #8928, #8880 ) ;
#2139=VERTEX_POINT ( 'NONE', #3786 ) ;
#2141=EDGE_CURVE ( 'NONE', #8924, #4397, #3522, .T. ) ;
#2144=DIRECTION ( 'NONE',  ( 0.000000000000000000, -1.000000000000000000, 0.000000000000000000 ) ) ;
#2150=CARTESIAN_POINT ( 'NONE',  ( -24.62111388750000174, 2.656249999044085097, -10.19839929293506131 ) ) ;
#2156=APPLICATION_CONTEXT ( 'automotive_design' ) ;
#2159=CARTESIAN_POINT ( 'NONE',  ( -10.19839929293507552, 3.906249999044085097, 24.62111388749999463 ) ) ;
#2170=CARTESIAN_POINT ( 'NONE',  ( 17.67766952966369232, 2.125000000000000000, -17.67766952966369232 ) ) ;
#2186=CARTESIAN_POINT ( 'NONE',  ( -25.00000000000000000, 3.437500000000000000, -10.35533905932738108 ) ) ;
#2189=EDGE_LOOP ( 'NONE', ( #6832, #8164, #8900, #9375, #8341 ) ) ;
#2192=DIRECTION ( 'NONE',  ( 0.000000000000000000, 0.000000000000000000, -1.000000000000000000 ) ) ;
#2206=CARTESIAN_POINT ( 'NONE',  ( -4.522825247065398226E-15, 1.968749999044084653, 24.62111388750000174 ) ) ;
#2210=ORIENTED_EDGE ( 'NONE', *, *, #10577, .F. ) ;
#2211=CARTESIAN_POINT ( 'NONE',  ( 25.00000000000000000, 4.674999998088169129, -10.35533905932737753 ) ) ;
#2224=( BOUNDED_CURVE ( )  B_SPLINE_CURVE ( 2, ( #8763, #1201, #2610, #6005, #9365, #1805, #1306, #4103, #10632 ),
 .UNSPECIFIED., .F., .F. ) 
 B_SPLINE_CURVE_WITH_KNOTS ( ( 3, 2, 2, 2, 3 ),
 ( 0.6500000000000000222, 0.6750000000000000444, 0.6999999999999999556, 0.7249999999999999778, 0.7500000000000000000 ),
 .UNSPECIFIED. ) 
 CURVE ( )  GEOMETRIC_REPRESENTATION_ITEM ( )  RATIONAL_B_SPLINE_CURVE ( ( 1.000000000000000000, 0.9238795325112867385, 1.000000000000000000, 0.9238795325112867385, 1.000000000000000000, 0.9238795325112867385, 1.000000000000000000, 0.9238795325112867385, 1.000000000000000000 ) ) 
 REPRESENTATION_ITEM ( '' )  );
#2243=( NAMED_UNIT ( * ) PLANE_ANGLE_UNIT ( ) SI_UNIT ( $, .RADIAN. ) );
#2250=EDGE_CURVE ( 'NONE', #5382, #57, #3190, .T. ) ;
#2260=ORIENTED_EDGE ( 'NONE', *, *, #318, .F. ) ;
#2262=CARTESIAN_POINT ( 'NONE',  ( -17.67766952966368876, 4.987499998088170017, -17.67766952966369232 ) ) ;
#2282=AXIS2_PLACEMENT_3D ( 'NONE', #6034, #8445, #1711 ) ;
#2285=CARTESIAN_POINT ( 'NONE',  ( 25.00000000000000000, 5.000000000000000000, 0.000000000000000000 ) ) ;
#2287=CARTESIAN_POINT ( 'NONE',  ( -24.62111388750000174, 2.718749999044084653, -3.015216831376932151E-15 ) ) ;
#2307=CARTESIAN_POINT ( 'NONE',  ( -4.592425496802574367E-15, 3.362499998088169129, 25.00000000000000000 ) ) ;
#2315=CARTESIAN_POINT ( 'NONE',  ( 1.507608415688466075E-15, 0.6437499990440845865, -24.62111388750000174 ) ) ;
#2316=DIRECTION ( 'NONE',  ( 0.000000000000000000, -1.000000000000000000, 0.000000000000000000 ) ) ;
#2340=CARTESIAN_POINT ( 'NONE',  ( -10.19839929293505776, 2.531249999044085097, -24.62111388750000174 ) ) ;
#2341=CARTESIAN_POINT ( 'NONE',  ( -4.592425496802574367E-15, 3.362499998088169129, 25.00000000000000000 ) ) ;
#2359=SURFACE_STYLE_USAGE ( .BOTH. , #1526 ) ;
#2365=FACE_OUTER_BOUND ( 'NONE', #270, .T. ) ;
#2371=CARTESIAN_POINT ( 'NONE',  ( 24.99999999999999289, 5.549999998088169129, 10.35533905932739529 ) ) ;
#2391=DIRECTION ( 'NONE',  ( 0.000000000000000000, 0.000000000000000000, -1.000000000000000000 ) ) ;
#2392=CARTESIAN_POINT ( 'NONE',  ( -24.62111388750000884, 3.781249999044084653, 10.19839929293505421 ) ) ;
#2401=CARTESIAN_POINT ( 'NONE',  ( 17.32475613793127422, 5.000000000000000000, 17.73196534595880536 ) ) ;
#2403=ORIENTED_EDGE ( 'NONE', *, *, #4857, .F. ) ;
#2408=CARTESIAN_POINT ( 'NONE',  ( 24.99999999999999289, 3.549999998088169573, 10.35533905932739529 ) ) ;
#2411=FACE_OUTER_BOUND ( 'NONE', #2628, .T. ) ;
#2417=CARTESIAN_POINT ( 'NONE',  ( -25.00000000000001421, 5.174999998088170017, 10.35533905932737397 ) ) ;
#2420=CIRCLE ( 'NONE', #10016, 27.91176187412963117 ) ;
#2433=ORIENTED_EDGE ( 'NONE', *, *, #317, .F. ) ;
#2439=CARTESIAN_POINT ( 'NONE',  ( 1.530808498934191521E-15, 4.862499998088169129, -25.00000000000000000 ) ) ;
#2441=CARTESIAN_POINT ( 'NONE',  ( 24.62111388750000174, 1.218749999044084431, 0.000000000000000000 ) ) ;
#2449=CARTESIAN_POINT ( 'NONE',  ( 0.000000000000000000, 0.000000000000000000, 0.000000000000000000 ) ) ;
#2450=CARTESIAN_POINT ( 'NONE',  ( 24.99999999999999289, 0.9375000000000000000, 10.35533905932739529 ) ) ;
#2452=CARTESIAN_POINT ( 'NONE',  ( 4.895565917430008795, 5.000000000000001776, 24.12949820052922334 ) ) ;
#2458=CYLINDRICAL_SURFACE ( 'NONE', #8971, 25.00000000000000000 ) ;
#2462=SHAPE_DEFINITION_REPRESENTATION ( #7769, #4232 ) ;
#2470=CARTESIAN_POINT ( 'NONE',  ( 10.19839929293505953, 4.581249999044083587, -24.62111388750000174 ) ) ;
#2477=CARTESIAN_POINT ( 'NONE',  ( 0.000000000000000000, -55.00000000000000000, 0.000000000000000000 ) ) ;
#2486=CARTESIAN_POINT ( 'NONE',  ( -4.149081428685724049, 5.000000000000003553, 24.37508152705383679 ) ) ;
#2488=CARTESIAN_POINT ( 'NONE',  ( -17.40975659021752975, 3.593749999044084653, -17.40975659021752975 ) ) ;
#2495=AXIS2_PLACEMENT_3D ( 'NONE', #5510, #8876, #7173 ) ;
#2504=CARTESIAN_POINT ( 'NONE',  ( 7.644054968599810707, 5.000000000000000000, 23.44899443080850787 ) ) ;
#2518=CIRCLE ( 'NONE', #3405, 27.91176187412963117 ) ;
#2523=EDGE_CURVE ( 'NONE', #1642, #8219, #1957, .T. ) ;
#2524=CARTESIAN_POINT ( 'NONE',  ( 24.62111388750000174, 3.393749999044084475, 0.000000000000000000 ) ) ;
#2539=CARTESIAN_POINT ( 'NONE',  ( -17.40975659021752975, 4.768749999044085364, -17.40975659021752975 ) ) ;
#2543=EDGE_CURVE ( 'NONE', #5838, #9967, #10850, .T. ) ;
#2544=CARTESIAN_POINT ( 'NONE',  ( -25.00000000000001066, 2.174999998088168685, 10.35533905932737397 ) ) ;
#2546=CARTESIAN_POINT ( 'NONE',  ( 25.00000000000000000, 0.06249999999999997224, -10.35533905932737753 ) ) ;
#2555=DIRECTION ( 'NONE',  ( 0.000000000000000000, -1.000000000000000000, 0.000000000000000000 ) ) ;
#2557=CARTESIAN_POINT ( 'NONE',  ( 24.81930730699091114, 5.000000000000000000, 2.826949417608202619 ) ) ;
#2564=( BOUNDED_CURVE ( )  B_SPLINE_CURVE ( 2, ( #2307, #5741, #1585, #2408, #3981, #5635, #7331, #8324, #8993 ),
 .UNSPECIFIED., .F., .F. ) 
 B_SPLINE_CURVE_WITH_KNOTS ( ( 3, 2, 2, 2, 3 ),
 ( 0.5500000000000000444, 0.5749999999999999556, 0.5999999999999999778, 0.6250000000000000000, 0.6500000000000000222 ),
 .UNSPECIFIED. ) 
 CURVE ( )  GEOMETRIC_REPRESENTATION_ITEM ( )  RATIONAL_B_SPLINE_CURVE ( ( 1.000000000000000000, 0.9238795325112867385, 1.000000000000000000, 0.9238795325112867385, 1.000000000000000000, 0.9238795325112867385, 1.000000000000000000, 0.9238795325112867385, 1.000000000000000000 ) ) 
 REPRESENTATION_ITEM ( '' )  );
#2572=VERTEX_POINT ( 'NONE', #8360 ) ;
#2574=CARTESIAN_POINT ( 'NONE',  ( 24.62111388750000174, 3.456249999044084920, -10.19839929293505776 ) ) ;
#2575=DIRECTION ( 'NONE',  ( 0.000000000000000000, -1.000000000000000000, 0.000000000000000000 ) ) ;
#2580=AXIS2_PLACEMENT_3D ( 'NONE', #5534, #7093, #8743 ) ;
#2581=CARTESIAN_POINT ( 'NONE',  ( 24.99999999999999289, 1.549999998088169129, 10.35533905932739529 ) ) ;
#2585=EDGE_CURVE ( 'NONE', #2663, #5323, #6852, .T. ) ;
#2594=CARTESIAN_POINT ( 'NONE',  ( -24.62111388750000884, 2.956249999044084475, 10.19839929293505421 ) ) ;
#2602=CARTESIAN_POINT ( 'NONE',  ( 25.00000000000000000, 1.062500000000000222, -10.35533905932737753 ) ) ;
#2610=CARTESIAN_POINT ( 'NONE',  ( -17.67766952966368876, 3.987499998088168685, -17.67766952966369232 ) ) ;
#2611=VERTEX_POINT ( 'NONE', #4399 ) ;
#2628=EDGE_LOOP ( 'NONE', ( #8081, #5108, #1233, #8278 ) ) ;
#2631=CARTESIAN_POINT ( 'NONE',  ( -17.40975659021752975, 0.7687499990440846975, -17.40975659021752975 ) ) ;
#2632=CARTESIAN_POINT ( 'NONE',  ( 24.62111388749999463, 3.331249999044084920, 10.19839929293507730 ) ) ;
#2637=FACE_OUTER_BOUND ( 'NONE', #3754, .T. ) ;
#2641=CARTESIAN_POINT ( 'NONE',  ( 10.35533905932738286, 2.424999998088169129, 24.99999999999999645 ) ) ;
#2643=CARTESIAN_POINT ( 'NONE',  ( 25.00000000000000000, 4.062500000000000000, -10.35533905932737753 ) ) ;
#2646=CARTESIAN_POINT ( 'NONE',  ( 10.19839929293505953, 2.581249999044084475, -24.62111388750000174 ) ) ;
#2658=CARTESIAN_POINT ( 'NONE',  ( 10.35533905932738286, 4.812500000000000888, 24.99999999999999645 ) ) ;
#2659=CARTESIAN_POINT ( 'NONE',  ( 1.530808498934191521E-15, 0.2500000000000000000, -25.00000000000000000 ) ) ;
#2661=ADVANCED_FACE ( 'NONE', ( #8754 ), #1243, .T. ) ;
#2663=VERTEX_POINT ( 'NONE', #1794 ) ;
#2683=CARTESIAN_POINT ( 'NONE',  ( -18.39893213276270956, 4.993656359492002039, -16.95640692656465731 ) ) ;
#2685=CARTESIAN_POINT ( 'NONE',  ( 1.507608415688466075E-15, 1.643749999044084475, -24.62111388750000174 ) ) ;
#2687=AXIS2_PLACEMENT_3D ( 'NONE', #10501, #8680, #1124 ) ;
#2695=CARTESIAN_POINT ( 'NONE',  ( 24.62111388749999463, 1.331249999044084475, 10.19839929293507730 ) ) ;
#2696=DIRECTION ( 'NONE',  ( 0.000000000000000000, 0.000000000000000000, -1.000000000000000000 ) ) ;
#2704=CARTESIAN_POINT ( 'NONE',  ( -17.67766952966369232, 2.237499998088169573, 17.67766952966368876 ) ) ;
#2707=CARTESIAN_POINT ( 'NONE',  ( 1.530808498934191521E-15, 3.250000000000000444, -25.00000000000000000 ) ) ;
#2709=ORIENTED_EDGE ( 'NONE', *, *, #6287, .F. ) ;
#2711=CARTESIAN_POINT ( 'NONE',  ( -24.62111388750000174, 4.831249999044085364, -10.19839929293506131 ) ) ;
#2712=CARTESIAN_POINT ( 'NONE',  ( 1.530808498934191521E-15, 0.2500000000000000000, -25.00000000000000000 ) ) ;
#2718=CARTESIAN_POINT ( 'NONE',  ( 10.35533905932737930, 0.1874999999999999722, -25.00000000000000000 ) ) ;
#2719=CARTESIAN_POINT ( 'NONE',  ( -4.592425496802574367E-15, 2.362499998088169129, 25.00000000000000000 ) ) ;
#2728=EDGE_LOOP ( 'NONE', ( #1524, #3074 ) ) ;
#2738=CARTESIAN_POINT ( 'NONE',  ( -4.592425496802574367E-15, 2.750000000000000000, 25.00000000000000000 ) ) ;
#2740=CARTESIAN_POINT ( 'NONE',  ( -24.62111388750000174, 1.893749999044084475, -3.015216831376932151E-15 ) ) ;
#2760=CARTESIAN_POINT ( 'NONE',  ( 1.530808498934191521E-15, 2.250000000000000444, -25.00000000000000000 ) ) ;
#2761=CARTESIAN_POINT ( 'NONE',  ( 17.40975659021752975, 2.518749999044084475, -17.40975659021752975 ) ) ;
#2767=CARTESIAN_POINT ( 'NONE',  ( 0.000000000000000000, -58.00000000000000000, 0.000000000000000000 ) ) ;
#2770=CARTESIAN_POINT ( 'NONE',  ( -24.62111388750000174, 4.656249999044085541, -10.19839929293506131 ) ) ;
#2772=ORIENTED_EDGE ( 'NONE', *, *, #317, .T. ) ;
#2793=CARTESIAN_POINT ( 'NONE',  ( -24.62111388750000884, 1.956249999044084698, 10.19839929293505421 ) ) ;
#2795=EDGE_CURVE ( 'NONE', #2980, #2038, #7977, .T. ) ;
#2803=CARTESIAN_POINT ( 'NONE',  ( 0.000000000000000000, 5.000000000000000000, 0.000000000000000000 ) ) ;
#2811=CARTESIAN_POINT ( 'NONE',  ( 24.62111388749999108, 4.156249999044084653, 10.19839929293507730 ) ) ;
#2820=CARTESIAN_POINT ( 'NONE',  ( 17.40975659021752975, 2.343749999044085097, -17.40975659021752975 ) ) ;
#2826=CARTESIAN_POINT ( 'NONE',  ( -25.00000000000001066, 2.562500000000000444, 10.35533905932737397 ) ) ;
#2837=FACE_OUTER_BOUND ( 'NONE', #137, .T. ) ;
#2839=ADVANCED_FACE ( 'NONE', ( #7617 ), #8220, .T. ) ;
#2848=CARTESIAN_POINT ( 'NONE',  ( -10.19839929293505776, 3.706249999044085808, -24.62111388750000174 ) ) ;
#2861=LINE ( 'NONE', #3706, #5351 ) ;
#2867=CARTESIAN_POINT ( 'NONE',  ( 1.507608415688466075E-15, 4.468749999044084653, -24.62111388750000174 ) ) ;
#2876=CARTESIAN_POINT ( 'NONE',  ( -24.62111388750000174, 2.656249999044085097, -10.19839929293506131 ) ) ;
#2883=DIRECTION ( 'NONE',  ( 0.000000000000000000, -1.000000000000000000, 0.000000000000000000 ) ) ;
#2885=VECTOR ( 'NONE', #9447, 1000.000000000000000 ) ;
#2886=VERTEX_POINT ( 'NONE', #5801 ) ;
#2904=CARTESIAN_POINT ( 'NONE',  ( -4.522825247065398226E-15, 5.143749999044084475, 24.62111388750000174 ) ) ;
#2911=ORIENTED_EDGE ( 'NONE', *, *, #4602, .F. ) ;
#2912=CARTESIAN_POINT ( 'NONE',  ( 10.19839929293506486, 4.031249999044083765, 24.62111388749999819 ) ) ;
#2918=DIRECTION ( 'NONE',  ( -0.000000000000000000, 1.000000000000000000, -0.000000000000000000 ) ) ;
#2919=CARTESIAN_POINT ( 'NONE',  ( -17.40975659021752975, 3.593749999044084653, -17.40975659021752975 ) ) ;
#2925=EDGE_CURVE ( 'NONE', #6596, #2139, #5480, .T. ) ;
#2929=CARTESIAN_POINT ( 'NONE',  ( 0.000000000000000000, -8.000000000000000000, 0.000000000000000000 ) ) ;
#2948=CARTESIAN_POINT ( 'NONE',  ( 0.000000000000000000, 5.000000000000000000, -25.00000000000000000 ) ) ;
#2953=ORIENTED_EDGE ( 'NONE', *, *, #6071, .F. ) ;
#2958=DIRECTION ( 'NONE',  ( 0.000000000000000000, -1.000000000000000000, 0.000000000000000000 ) ) ;
#2961=ORIENTED_EDGE ( 'NONE', *, *, #10313, .T. ) ;
#2962=CARTESIAN_POINT ( 'NONE',  ( -17.40975659021753330, 1.843749999044084653, 17.40975659021752975 ) ) ;
#2969=DIRECTION ( 'NONE',  ( 0.000000000000000000, 0.000000000000000000, 1.000000000000000000 ) ) ;
#2970=CARTESIAN_POINT ( 'NONE',  ( 24.62111388750000174, 1.218749999044084431, 0.000000000000000000 ) ) ;
#2980=VERTEX_POINT ( 'NONE', #7510 ) ;
#2983=ORIENTED_EDGE ( 'NONE', *, *, #2250, .T. ) ;
#2988=( BOUNDED_CURVE ( )  B_SPLINE_CURVE ( 2, ( #3954, #10684, #7305, #3093, #568, #8116, #9625, #2100, #4712 ),
 .UNSPECIFIED., .F., .F. ) 
 B_SPLINE_CURVE_WITH_KNOTS ( ( 3, 2, 2, 2, 3 ),
 ( 0.7500000000000000000, 0.7750000000000000222, 0.8000000000000000444, 0.8250000000000000666, 0.8500000000000000888 ),
 .UNSPECIFIED. ) 
 CURVE ( )  GEOMETRIC_REPRESENTATION_ITEM ( )  RATIONAL_B_SPLINE_CURVE ( ( 1.000000000000000000, 0.9238795325112867385, 1.000000000000000000, 0.9238795325112867385, 1.000000000000000000, 0.9238795325112867385, 1.000000000000000000, 0.9238795325112864054, 1.000000000000000444 ) ) 
 REPRESENTATION_ITEM ( '' )  );
#3002=FACE_OUTER_BOUND ( 'NONE', #6915, .T. ) ;
#3020=CARTESIAN_POINT ( 'NONE',  ( -17.40975659021752975, 2.593749999044084653, -17.40975659021752975 ) ) ;
#3028=CARTESIAN_POINT ( 'NONE',  ( -10.35533905932739174, 4.299999998088169129, 24.99999999999999289 ) ) ;
#3029=CARTESIAN_POINT ( 'NONE',  ( -4.522825247065398226E-15, 4.968749999044083765, 24.62111388750000174 ) ) ;
#3042=CARTESIAN_POINT ( 'NONE',  ( -17.67766952966369232, 0.6250000000000000000, 17.67766952966368876 ) ) ;
#3054=( BOUNDED_CURVE ( )  B_SPLINE_CURVE ( 2, ( #9773, #10451, #1330, #6368, #8061 ),
 .UNSPECIFIED., .F., .F. ) 
 B_SPLINE_CURVE_WITH_KNOTS ( ( 3, 2, 3 ),
 ( 0.000000000000000000, 0.02500000000000000486, 0.05000000000000000971 ),
 .UNSPECIFIED. ) 
 CURVE ( )  GEOMETRIC_REPRESENTATION_ITEM ( )  RATIONAL_B_SPLINE_CURVE ( ( 1.000000000000000000, 0.9238795325112867385, 1.000000000000000000, 0.9238795325112867385, 1.000000000000000000 ) ) 
 REPRESENTATION_ITEM ( '' )  );
#3061=CARTESIAN_POINT ( 'NONE',  ( 25.00000000000000000, 1.062500000000000222, -10.35533905932737753 ) ) ;
#3070=ORIENTED_EDGE ( 'NONE', *, *, #4644, .T. ) ;
#3074=ORIENTED_EDGE ( 'NONE', *, *, #8684, .T. ) ;
#3079=EDGE_LOOP ( 'NONE', ( #4222, #5495, #8353, #1863 ) ) ;
#3081=CARTESIAN_POINT ( 'NONE',  ( 1.530808498934191521E-15, 2.862499998088169573, -25.00000000000000000 ) ) ;
#3093=CARTESIAN_POINT ( 'NONE',  ( 24.99999999999999289, 3.937500000000000000, 10.35533905932739529 ) ) ;
#3098=CARTESIAN_POINT ( 'NONE',  ( -17.40975659021752975, 0.5937499990440846531, -17.40975659021752975 ) ) ;
#3129=EDGE_CURVE ( 'NONE', #2572, #3847, #8119, .T. ) ;
#3130=CARTESIAN_POINT ( 'NONE',  ( 24.62111388750000174, 0.3937499990440845310, 0.000000000000000000 ) ) ;
#3135=DIRECTION ( 'NONE',  ( -0.000000000000000000, 1.000000000000000000, -0.000000000000000000 ) ) ;
#3142=( BOUNDED_CURVE ( )  B_SPLINE_CURVE ( 2, ( #7724, #8430, #9313, #5137, #3579, #9253, #6020, #1646, #6843 ),
 .UNSPECIFIED., .F., .F. ) 
 B_SPLINE_CURVE_WITH_KNOTS ( ( 3, 2, 2, 2, 3 ),
 ( 0.8500000000000000888, 0.8750000000000001110, 0.9000000000000001332, 0.9250000000000001554, 0.9500000000000000666 ),
 .UNSPECIFIED. ) 
 CURVE ( )  GEOMETRIC_REPRESENTATION_ITEM ( )  RATIONAL_B_SPLINE_CURVE ( ( 0.9999999999999996669, 0.9238795325112870716, 1.000000000000000000, 0.9238795325112867385, 1.000000000000000000, 0.9238795325112867385, 1.000000000000000000, 0.9238795325112864054, 1.000000000000000444 ) ) 
 REPRESENTATION_ITEM ( '' )  );
#3151=DIRECTION ( 'NONE',  ( -0.8660254037844402619, -0.4999999999999971134, 0.000000000000000000 ) ) ;
#3152=CARTESIAN_POINT ( 'NONE',  ( 10.19839929293505953, 1.406249999044084653, -24.62111388750000174 ) ) ;
#3153=CARTESIAN_POINT ( 'NONE',  ( -17.67766952966369232, 3.625000000000000000, 17.67766952966368876 ) ) ;
#3174=ORIENTED_EDGE ( 'NONE', *, *, #318, .T. ) ;
#3177=ORIENTED_EDGE ( 'NONE', *, *, #5396, .F. ) ;
#3181=CARTESIAN_POINT ( 'NONE',  ( 24.99999999999999289, 3.549999998088169573, 10.35533905932739529 ) ) ;
#3182=CARTESIAN_POINT ( 'NONE',  ( 17.40975659021752620, 5.093749999044084653, 17.40975659021753330 ) ) ;
#3190=LINE ( 'NONE', #3421, #9162 ) ;
#3194=ORIENTED_EDGE ( 'NONE', *, *, #1096, .T. ) ;
#3206=CARTESIAN_POINT ( 'NONE',  ( 10.19839929293505953, 2.406249999044085541, -24.62111388750000174 ) ) ;
#3208=AXIS2_PLACEMENT_3D ( 'NONE', #6134, #8047, #481 ) ;
#3216=DIRECTION ( 'NONE',  ( 0.000000000000000000, -1.000000000000000000, 0.000000000000000000 ) ) ;
#3217=CARTESIAN_POINT ( 'NONE',  ( 0.000000000000000000, -0.5289809421253948152, 0.000000000000000000 ) ) ;
#3224=CARTESIAN_POINT ( 'NONE',  ( 1.507608415688466075E-15, 0.6437499990440845865, -24.62111388750000174 ) ) ;
#3232=CARTESIAN_POINT ( 'NONE',  ( 10.35533905932738286, 5.424999998088169129, 24.99999999999999645 ) ) ;
#3238=DIRECTION ( 'NONE',  ( 0.000000000000000000, 0.000000000000000000, -1.000000000000000000 ) ) ;
#3248=EDGE_CURVE ( 'NONE', #1367, #2572, #6195, .T. ) ;
#3257=CARTESIAN_POINT ( 'NONE',  ( -17.40975659021753330, 2.843749999044085097, 17.40975659021752975 ) ) ;
#3269=( BOUNDED_CURVE ( )  B_SPLINE_CURVE ( 2, ( #764, #6911, #10265, #2683, #8429 ),
 .UNSPECIFIED., .F., .F. ) 
 B_SPLINE_CURVE_WITH_KNOTS ( ( 3, 2, 3 ),
 ( 0.8500000000000000888, 0.8750000000000000000, 0.8776439810613864134 ),
 .UNSPECIFIED. ) 
 CURVE ( )  GEOMETRIC_REPRESENTATION_ITEM ( )  RATIONAL_B_SPLINE_CURVE ( ( 0.9999999999999996669, 0.9238795325112870716, 1.000000000000000000, 0.9919495570230385528, 0.9856019315474255915 ) ) 
 REPRESENTATION_ITEM ( '' )  );
#3271=CARTESIAN_POINT ( 'NONE',  ( 6.281342968951019401, 5.000000000000000888, 23.83348803927349024 ) ) ;
#3283=ORIENTED_EDGE ( 'NONE', *, *, #5539, .F. ) ;
#3289=CARTESIAN_POINT ( 'NONE',  ( 24.62111388750000174, 4.393749999044084475, 0.000000000000000000 ) ) ;
#3310=CARTESIAN_POINT ( 'NONE',  ( -6.389531198409865276, 5.000000000000000000, 23.88578866465264383 ) ) ;
#3312=CARTESIAN_POINT ( 'NONE',  ( 10.19839929293505953, 3.406249999044085097, -24.62111388750000174 ) ) ;
#3313=CARTESIAN_POINT ( 'NONE',  ( 0.000000000000000000, 5.000000000000000000, 0.000000000000000000 ) ) ;
#3316=EDGE_LOOP ( 'NONE', ( #1612, #10159, #3174, #6497 ) ) ;
#3326=DIRECTION ( 'NONE',  ( 0.000000000000000000, -1.000000000000000000, 0.000000000000000000 ) ) ;
#3334=CONICAL_SURFACE ( 'NONE', #9173, 22.18092213764227694, 0.3490658503988666728 ) ;
#3340=MANIFOLD_SOLID_BREP ( 'Cavity1', #322 ) ;
#3349=CARTESIAN_POINT ( 'NONE',  ( 17.40975659021752975, 2.518749999044084475, -17.40975659021752975 ) ) ;
#3367=CARTESIAN_POINT ( 'NONE',  ( -17.40975659021752975, 0.5937499990440846531, -17.40975659021752975 ) ) ;
#3376=VERTEX_POINT ( 'NONE', #8106 ) ;
#3386=CARTESIAN_POINT ( 'NONE',  ( -4.592425496802574367E-15, 1.750000000000000000, 25.00000000000000000 ) ) ;
#3405=AXIS2_PLACEMENT_3D ( 'NONE', #3802, #7175, #10538 ) ;
#3406=DIRECTION ( 'NONE',  ( -0.000000000000000000, 1.000000000000000000, -0.000000000000000000 ) ) ;
#3410=CARTESIAN_POINT ( 'NONE',  ( -4.522825247065398226E-15, 1.143749999044084475, 24.62111388750000174 ) ) ;
#3411=CARTESIAN_POINT ( 'NONE',  ( 1.507608415688466075E-15, 2.643749999044084920, -24.62111388750000174 ) ) ;
#3419=CARTESIAN_POINT ( 'NONE',  ( 1.530808498934191521E-15, 0.8624999980881691286, -25.00000000000000000 ) ) ;
#3421=CARTESIAN_POINT ( 'NONE',  ( 0.000000000000000000, 5.000000000000000000, -25.00000000000000000 ) ) ;
#3427=CARTESIAN_POINT ( 'NONE',  ( -4.522825247065398226E-15, 0.9687499990440845421, 24.62111388750000174 ) ) ;
#3431=DIRECTION ( 'NONE',  ( 0.000000000000000000, 0.000000000000000000, 1.000000000000000000 ) ) ;
#3433=CARTESIAN_POINT ( 'NONE',  ( -10.35533905932739174, 2.299999998088169129, 24.99999999999999289 ) ) ;
#3436=CARTESIAN_POINT ( 'NONE',  ( -4.592425496802574367E-15, 0.7500000000000000000, 25.00000000000000000 ) ) ;
#3442=DIRECTION ( 'NONE',  ( 0.000000000000000000, -1.000000000000000000, 0.000000000000000000 ) ) ;
#3463=EDGE_CURVE ( 'NONE', #2038, #6538, #3269, .T. ) ;
#3465=CARTESIAN_POINT ( 'NONE',  ( 24.62111388750000174, 0.3937499990440845865, 0.000000000000000000 ) ) ;
#3466=CARTESIAN_POINT ( 'NONE',  ( -17.40975659021752975, 2.768749999044084475, -17.40975659021752975 ) ) ;
#3476=CARTESIAN_POINT ( 'NONE',  ( -25.00000000000001421, 2.174999998088169573, 10.35533905932737397 ) ) ;
#3478=CARTESIAN_POINT ( 'NONE',  ( -10.35533905932737575, 4.312500000000000888, -25.00000000000000000 ) ) ;
#3486=CARTESIAN_POINT ( 'NONE',  ( 24.62111388750000174, 0.2812499990440845976, -10.19839929293505776 ) ) ;
#3498=CARTESIAN_POINT ( 'NONE',  ( 10.35533905932737930, 1.187500000000000444, -25.00000000000000000 ) ) ;
#3507=CARTESIAN_POINT ( 'NONE',  ( 24.99999999999999289, 1.937500000000000000, 10.35533905932739529 ) ) ;
#3518=CARTESIAN_POINT ( 'NONE',  ( 24.62111388750000174, 2.456249999044084475, -10.19839929293505776 ) ) ;
#3522=CIRCLE ( 'NONE', #10411, 27.91176187412962761 ) ;
#3525=AXIS2_PLACEMENT_3D ( 'NONE', #6846, #9445, #10268 ) ;
#3527=CARTESIAN_POINT ( 'NONE',  ( -24.62111388750000174, 2.831249999044084475, -10.19839929293506131 ) ) ;
#3528=CARTESIAN_POINT ( 'NONE',  ( 0.000000000000000000, -58.00000000000000000, 0.000000000000000000 ) ) ;
#3534=CARTESIAN_POINT ( 'NONE',  ( 1.507608415688466075E-15, 0.4687499990440845421, -24.62111388750000174 ) ) ;
#3536=CARTESIAN_POINT ( 'NONE',  ( -4.592425496802574367E-15, 2.362499998088169129, 25.00000000000000000 ) ) ;
#3544=CARTESIAN_POINT ( 'NONE',  ( -17.40975659021753330, 3.018749999044084475, 17.40975659021752975 ) ) ;
#3555=CARTESIAN_POINT ( 'NONE',  ( -25.00000000000001421, 0.5625000000000001110, 10.35533905932737397 ) ) ;
#3557=ORIENTED_EDGE ( 'NONE', *, *, #738, .T. ) ;
#3579=CARTESIAN_POINT ( 'NONE',  ( -25.00000000000000000, 4.500000000000000888, -3.061616997868383043E-15 ) ) ;
#3580=CARTESIAN_POINT ( 'NONE',  ( 1.507608415688466075E-15, 3.643749999044084920, -24.62111388750000174 ) ) ;
#3588=AXIS2_PLACEMENT_3D ( 'NONE', #10317, #9648, #4477 ) ;
#3591=CIRCLE ( 'NONE', #10653, 22.00000000000000355 ) ;
#3592=CARTESIAN_POINT ( 'NONE',  ( 1.530808498934191521E-15, 0.8624999980881691286, -25.00000000000000000 ) ) ;
#3599=CARTESIAN_POINT ( 'NONE',  ( 10.35533905932738286, 2.812500000000000000, 24.99999999999999645 ) ) ;
#3604=CARTESIAN_POINT ( 'NONE',  ( 10.19839929293506486, 5.206249999044084475, 24.62111388749999819 ) ) ;
#3614=VERTEX_POINT ( 'NONE', #9744 ) ;
#3619=LINE ( 'NONE', #8648, #7036 ) ;
#3622=ORIENTED_EDGE ( 'NONE', *, *, #7467, .F. ) ;
#3624=EDGE_CURVE ( 'NONE', #10065, #5382, #7449, .T. ) ;
#3635=CARTESIAN_POINT ( 'NONE',  ( 25.00000000000000000, 3.000000000000000000, 0.000000000000000000 ) ) ;
#3637=CARTESIAN_POINT ( 'NONE',  ( -17.40975659021753330, 2.018749999044084475, 17.40975659021752975 ) ) ;
#3658=CARTESIAN_POINT ( 'NONE',  ( -17.40975659021753330, 2.018749999044084475, 17.40975659021752975 ) ) ;
#3661=CARTESIAN_POINT ( 'NONE',  ( 10.19839929293506486, 4.031249999044083765, 24.62111388749999819 ) ) ;
#3668=DIRECTION ( 'NONE',  ( 0.000000000000000000, 0.000000000000000000, 1.000000000000000000 ) ) ;
#3672=ORIENTED_EDGE ( 'NONE', *, *, #5396, .T. ) ;
#3673=AXIS2_PLACEMENT_3D ( 'NONE', #1200, #7985, #7111 ) ;
#3676=VERTEX_POINT ( 'NONE', #1454 ) ;
#3684=ADVANCED_FACE ( 'NONE', ( #5815 ), #7393, .F. ) ;
#3692=CARTESIAN_POINT ( 'NONE',  ( 24.62111388750000174, 3.456249999044084920, -10.19839929293505776 ) ) ;
#3702=CARTESIAN_POINT ( 'NONE',  ( -17.40975659021753330, 5.018749999044084475, 17.40975659021752975 ) ) ;
#3704=CARTESIAN_POINT ( 'NONE',  ( -22.42673455797375937, 5.000000000000000000, 10.41080002251884018 ) ) ;
#3706=CARTESIAN_POINT ( 'NONE',  ( 3.061616997868383043E-15, 5.000000000000000000, 25.00000000000000000 ) ) ;
#3711=CARTESIAN_POINT ( 'NONE',  ( 1.507608415688466075E-15, 2.468749999044085097, -24.62111388750000174 ) ) ;
#3721=CARTESIAN_POINT ( 'NONE',  ( 24.62111388750000174, 1.281249999044084653, -10.19839929293505776 ) ) ;
#3726=CARTESIAN_POINT ( 'NONE',  ( 2.694222958124177204E-15, 5.000000000000000000, 22.00000000000000355 ) ) ;
#3731=AXIS2_PLACEMENT_3D ( 'NONE', #4944, #5664, #5759 ) ;
#3732=CARTESIAN_POINT ( 'NONE',  ( 3.061616997868383043E-15, 0.000000000000000000, 25.00000000000000000 ) ) ;
#3745=CARTESIAN_POINT ( 'NONE',  ( 24.62111388749999108, 4.331249999044084475, 10.19839929293507730 ) ) ;
#3754=EDGE_LOOP ( 'NONE', ( #9740, #10701, #2911, #9106, #3070, #10295 ) ) ;
#3759=CARTESIAN_POINT ( 'NONE',  ( -24.62111388750000884, 4.956249999044084475, 10.19839929293505421 ) ) ;
#3765=FACE_OUTER_BOUND ( 'NONE', #2728, .T. ) ;
#3768=CARTESIAN_POINT ( 'NONE',  ( -24.62111388750000884, 4.781249999044083765, 10.19839929293505421 ) ) ;
#3778=CARTESIAN_POINT ( 'NONE',  ( 24.62111388749999463, 2.156249999044085097, 10.19839929293507730 ) ) ;
#3780=AXIS2_PLACEMENT_3D ( 'NONE', #10812, #3216, #2192 ) ;
#3786=CARTESIAN_POINT ( 'NONE',  ( 25.00000000000000000, -2.710505431213761085E-17, 0.000000000000000000 ) ) ;
#3802=CARTESIAN_POINT ( 'NONE',  ( 0.000000000000000000, -55.00000000000000000, 0.000000000000000000 ) ) ;
#3808=CARTESIAN_POINT ( 'NONE',  ( -23.76354281994116846, 5.000000000000000000, -7.534344838453043813 ) ) ;
#3815=CARTESIAN_POINT ( 'NONE',  ( 10.19839929293506486, 2.031249999044084653, 24.62111388749999819 ) ) ;
#3825=CARTESIAN_POINT ( 'NONE',  ( 17.40975659021752620, 1.093749999044084653, 17.40975659021753330 ) ) ;
#3831=CARTESIAN_POINT ( 'NONE',  ( 0.000000000000000000, -55.00000000000000000, 27.91176187412963117 ) ) ;
#3832=DIRECTION ( 'NONE',  ( 0.000000000000000000, -1.000000000000000000, 0.000000000000000000 ) ) ;
#3839=VECTOR ( 'NONE', #8168, 1000.000000000000000 ) ;
#3844=LINE ( 'NONE', #5723, #7625 ) ;
#3847=VERTEX_POINT ( 'NONE', #6927 ) ;
#3867=CARTESIAN_POINT ( 'NONE',  ( 25.00000000000000000, 2.674999998088169573, -10.35533905932737753 ) ) ;
#3869=CARTESIAN_POINT ( 'NONE',  ( 17.40975659021752975, 1.343749999044084653, -17.40975659021752975 ) ) ;
#3871=EDGE_LOOP ( 'NONE', ( #9480, #10454, #7966, #4729 ) ) ;
#3874=CARTESIAN_POINT ( 'NONE',  ( 10.19839929293506486, 3.031249999044084653, 24.62111388749999819 ) ) ;
#3877=ADVANCED_FACE ( 'NONE', ( #2637 ), #4260, .T. ) ;
#3890=CARTESIAN_POINT ( 'NONE',  ( 1.530808498934191521E-15, 0.2500000000000000000, -25.00000000000000000 ) ) ;
#3899=CYLINDRICAL_SURFACE ( 'NONE', #9046, 25.00000000000000000 ) ;
#3911=CARTESIAN_POINT ( 'NONE',  ( 0.000000000000000000, -58.00000000000000000, 0.000000000000000000 ) ) ;
#3919=AXIS2_PLACEMENT_3D ( 'NONE', #4625, #2883, #6278 ) ;
#3920=( LENGTH_UNIT ( ) NAMED_UNIT ( * ) SI_UNIT ( .MILLI., .METRE. ) );
#3928=CARTESIAN_POINT ( 'NONE',  ( -24.62111388750000174, 3.656249999044084653, -10.19839929293506131 ) ) ;
#3936=CARTESIAN_POINT ( 'NONE',  ( 17.67766952966369232, 3.737499998088169573, -17.67766952966369232 ) ) ;
#3954=CARTESIAN_POINT ( 'NONE',  ( -4.592425496802574367E-15, 3.750000000000000000, 25.00000000000000000 ) ) ;
#3969=CARTESIAN_POINT ( 'NONE',  ( 1.530808498934191521E-15, 0.8624999980881691286, -25.00000000000000000 ) ) ;
#3981=CARTESIAN_POINT ( 'NONE',  ( 25.00000000000000000, 3.612499998088169129, 0.000000000000000000 ) ) ;
#3989=EDGE_CURVE ( 'NONE', #4764, #3676, #7964, .T. ) ;
#3990=CARTESIAN_POINT ( 'NONE',  ( 25.00000000000000000, 5.612499998088169129, 0.000000000000000000 ) ) ;
#3999=EDGE_LOOP ( 'NONE', ( #1105, #2772, #4507, #747, #6795 ) ) ;
#4002=ORIENTED_EDGE ( 'NONE', *, *, #7682, .T. ) ;
#4008=CARTESIAN_POINT ( 'NONE',  ( -10.19839929293505776, 1.531249999044084653, -24.62111388750000174 ) ) ;
#4015=CIRCLE ( 'NONE', #3673, 2.999999999999999112 ) ;
#4018=CARTESIAN_POINT ( 'NONE',  ( 17.67766952966369232, 0.7374999980881691286, -17.67766952966369232 ) ) ;
#4021=CARTESIAN_POINT ( 'NONE',  ( 1.530808498934191521E-15, 1.250000000000000000, -25.00000000000000000 ) ) ;
#4042=CARTESIAN_POINT ( 'NONE',  ( 17.40975659021752620, 1.268749999044084475, 17.40975659021753330 ) ) ;
#4043=DIRECTION ( 'NONE',  ( 0.000000000000000000, 0.000000000000000000, -1.000000000000000000 ) ) ;
#4061=DIRECTION ( 'NONE',  ( 0.000000000000000000, -1.000000000000000000, 0.000000000000000000 ) ) ;
#4062=DIRECTION ( 'NONE',  ( 0.000000000000000000, 0.000000000000000000, -1.000000000000000000 ) ) ;
#4063=CARTESIAN_POINT ( 'NONE',  ( 17.40975659021752620, 1.093749999044084653, 17.40975659021753330 ) ) ;
#4064=DIRECTION ( 'NONE',  ( 0.000000000000000000, -1.000000000000000000, 0.000000000000000000 ) ) ;
#4083=CARTESIAN_POINT ( 'NONE',  ( -24.62111388750000174, 0.8312499990440843645, -10.19839929293506131 ) ) ;
#4097=CARTESIAN_POINT ( 'NONE',  ( -4.592425496802574367E-15, 4.362499998088169129, 25.00000000000000000 ) ) ;
#4103=CARTESIAN_POINT ( 'NONE',  ( -10.35533905932739174, 4.299999998088169129, 24.99999999999999289 ) ) ;
#4111=EDGE_CURVE ( 'NONE', #9754, #2886, #2564, .T. ) ;
#4122=CARTESIAN_POINT ( 'NONE',  ( -24.62111388750000174, 0.6562499990440846531, -10.19839929293506131 ) ) ;
#4149=CARTESIAN_POINT ( 'NONE',  ( 10.19839929293506486, 1.206249999044084698, 24.62111388749999819 ) ) ;
#4153=ORIENTED_EDGE ( 'NONE', *, *, #8898, .T. ) ;
#4168=CARTESIAN_POINT ( 'NONE',  ( 4.895565917430008795, 5.000000000000001776, 24.12949820052922334 ) ) ;
#4170=CARTESIAN_POINT ( 'NONE',  ( -24.62111388750000884, 2.781249999044085541, 10.19839929293505421 ) ) ;
#4180=CARTESIAN_POINT ( 'NONE',  ( 0.000000000000000000, 5.000000000000000000, 0.000000000000000000 ) ) ;
#4181=CARTESIAN_POINT ( 'NONE',  ( 24.72166399154381011, 4.999999999999999112, 3.527620825298249052 ) ) ;
#4198=CARTESIAN_POINT ( 'NONE',  ( -4.522825247065398226E-15, 2.143749999044084920, 24.62111388750000174 ) ) ;
#4213=CARTESIAN_POINT ( 'NONE',  ( 24.62111388750000174, 4.393749999044085364, 0.000000000000000000 ) ) ;
#4217=CARTESIAN_POINT ( 'NONE',  ( -4.592425496802574367E-15, 2.362499998088169129, 25.00000000000000000 ) ) ;
#4219=CARTESIAN_POINT ( 'NONE',  ( 10.35533905932738286, 4.424999998088169129, 24.99999999999999645 ) ) ;
#4220=CARTESIAN_POINT ( 'NONE',  ( 17.67766952966369232, 1.125000000000000222, -17.67766952966369232 ) ) ;
#4222=ORIENTED_EDGE ( 'NONE', *, *, #3624, .F. ) ;
#4232=SHAPE_REPRESENTATION ( 'Lower Catch Container', ( #7040 ), #8059 ) ;
#4235=CARTESIAN_POINT ( 'NONE',  ( 17.67766952966368521, 4.875000000000000000, 17.67766952966369232 ) ) ;
#4249=ADVANCED_FACE ( 'NONE', ( #8490 ), #825, .T. ) ;
#4255=CARTESIAN_POINT ( 'NONE',  ( -24.62111388750000174, 0.8312499990440845865, -10.19839929293506131 ) ) ;
#4256=CARTESIAN_POINT ( 'NONE',  ( 17.40975659021752620, 2.268749999044084475, 17.40975659021753330 ) ) ;
#4260=CYLINDRICAL_SURFACE ( 'NONE', #2282, 25.00000000000000000 ) ;
#4271=CARTESIAN_POINT ( 'NONE',  ( -17.40975659021753330, 4.018749999044084475, 17.40975659021752975 ) ) ;
#4277=ORIENTED_EDGE ( 'NONE', *, *, #7935, .T. ) ;
#4280=CARTESIAN_POINT ( 'NONE',  ( -17.67766952966368876, 1.987499998088169129, -17.67766952966369232 ) ) ;
#4281=CARTESIAN_POINT ( 'NONE',  ( 17.67766952966369232, 4.737499998088169129, -17.67766952966369232 ) ) ;
#4282=CARTESIAN_POINT ( 'NONE',  ( 17.67766952966368521, 0.8750000000000000000, 17.67766952966369232 ) ) ;
#4283=CARTESIAN_POINT ( 'NONE',  ( -10.35533905932737575, 2.924999998088169129, -25.00000000000000000 ) ) ;
#4294=CARTESIAN_POINT ( 'NONE',  ( 10.35533905932737930, 2.187500000000000444, -25.00000000000000000 ) ) ;
#4307=CARTESIAN_POINT ( 'NONE',  ( 24.62111388750000174, 0.3937499990440845310, 0.000000000000000000 ) ) ;
#4316=CARTESIAN_POINT ( 'NONE',  ( 1.507608415688466075E-15, 0.6437499990440845865, -24.62111388750000174 ) ) ;
#4317=CARTESIAN_POINT ( 'NONE',  ( 10.19839929293506486, 2.206249999044084920, 24.62111388749999819 ) ) ;
#4327=CARTESIAN_POINT ( 'NONE',  ( 10.35533905932737930, 4.187500000000000000, -25.00000000000000000 ) ) ;
#4333=CARTESIAN_POINT ( 'NONE',  ( -24.62111388750000174, 4.893749999044085364, -3.015216831376932151E-15 ) ) ;
#4338=CARTESIAN_POINT ( 'NONE',  ( 0.000000000000000000, -55.00000000000000000, 0.000000000000000000 ) ) ;
#4351=B_SPLINE_CURVE_WITH_KNOTS ( 'NONE', 3,
 ( #10145, #1639, #9371, #2557, #4181, #7545, #7661, #10927, #9307, #8542, #10873, #10200, #5197, #1751, #9975, #2401, #6730, #9195, #5781, #9146, #929, #1574, #8313, #7493, #2504, #3271, #6671, #2452 ),
 .UNSPECIFIED., .F., .F.,
 ( 4, 2, 2, 2, 2, 2, 2, 2, 2, 2, 2, 2, 2, 4 ),
 ( 0.000000000000000000, 0.002127673191709734957, 0.004255346383419469913, 0.008510692766838939827, 0.01063836595854867478, 0.01276603915025841147, 0.01702138553367788312, 0.01914905872538762502, 0.02127673191709736691, 0.02553207830051684377, 0.02765975149222657872, 0.02978742468393631368, 0.03191509787564604517, 0.03404277106735578012 ),
 .UNSPECIFIED. ) ;
#4357=ADVANCED_FACE ( 'NONE', ( #6796 ), #9315, .F. ) ;
#4360=CARTESIAN_POINT ( 'NONE',  ( 10.19839929293505953, 4.581249999044083587, -24.62111388750000174 ) ) ;
#4370=CARTESIAN_POINT ( 'NONE',  ( -24.62111388750000174, 0.8937499990440845865, -3.015216831376932151E-15 ) ) ;
#4371=CARTESIAN_POINT ( 'NONE',  ( 24.62111388750000174, 2.393749999044084475, 0.000000000000000000 ) ) ;
#4381=CARTESIAN_POINT ( 'NONE',  ( -19.39162934935757931, 5.000000000000000888, 15.17115553405142947 ) ) ;
#4382=CARTESIAN_POINT ( 'NONE',  ( 17.67766952966368521, 2.487499998088169129, 17.67766952966369232 ) ) ;
#4384=CARTESIAN_POINT ( 'NONE',  ( 17.67766952966369232, 3.125000000000000000, -17.67766952966369232 ) ) ;
#4390=CARTESIAN_POINT ( 'NONE',  ( 24.62111388750000174, 2.456249999044084475, -10.19839929293505776 ) ) ;
#4397=VERTEX_POINT ( 'NONE', #6974 ) ;
#4399=CARTESIAN_POINT ( 'NONE',  ( -4.592425496802574367E-15, 4.362499998088169129, 25.00000000000000000 ) ) ;
#4404=CARTESIAN_POINT ( 'NONE',  ( 10.19839929293505953, 4.406249999044084653, -24.62111388750000174 ) ) ;
#4420=PRODUCT ( 'Lower Catch Container', 'Lower Catch Container', '', ( #9817 ) ) ;
#4423=CARTESIAN_POINT ( 'NONE',  ( -10.19839929293505776, 4.706249999044084475, -24.62111388750000174 ) ) ;
#4438=CARTESIAN_POINT ( 'NONE',  ( 0.000000000000000000, 5.000000000000000000, 0.000000000000000000 ) ) ;
#4441=SURFACE_STYLE_USAGE ( .BOTH. , #10220 ) ;
#4445=CARTESIAN_POINT ( 'NONE',  ( -17.67766952966369232, 3.625000000000000000, 17.67766952966368876 ) ) ;
#4448=( BOUNDED_CURVE ( )  B_SPLINE_CURVE ( 2, ( #8681, #5221, #7803, #172, #3534, #9460, #1892, #237, #1126, #5763, #289, #7037, #10396, #9128, #7479, #7092, #1329, #547, #3869, #9675, #498, #9568, #2010, #6209, #7232, #6367, #2962, #5428, #2206, #3815, #4611, #394, #8060, #7967, #9725, #1375, #3711, #10608, #3020, #2150, #4760, #9623, #6421, #9772, #5385, #8841, #1282, #5533, #8896, #5584, #6309, #8943, #10450, #6264, #8115, #3928, #2099, #7144, #10503, #10553, #344, #2912, #7288, #2811, #7187, #449, #8742, #1181, #2867, #1230, #8790, #4559, #2054, #3768, #7916, #5476, #4665, #8017, #4711 ),
 .UNSPECIFIED., .F., .F. ) 
 B_SPLINE_CURVE_WITH_KNOTS ( ( 3, 2, 2, 2, 2, 2, 2, 2, 2, 2, 2, 2, 2, 2, 2, 2, 2, 2, 2, 2, 2, 2, 2, 2, 2, 2, 2, 2, 2, 2, 2, 2, 2, 2, 2, 2, 2, 2, 2, 3 ),
 ( 0.000000000000000000, 0.02500000000000000139, 0.05000000000000000278, 0.07499999999999999722, 0.1000000000000000056, 0.1250000000000000000, 0.1499999999999999944, 0.1749999999999999889, 0.2000000000000000111, 0.2250000000000000056, 0.2500000000000000000, 0.2750000000000000222, 0.2999999999999999889, 0.3250000000000000111, 0.3499999999999999778, 0.3750000000000000000, 0.4000000000000000222, 0.4249999999999999889, 0.4500000000000000111, 0.4749999999999999778, 0.5000000000000000000, 0.5250000000000000222, 0.5500000000000000444, 0.5749999999999999556, 0.5999999999999999778, 0.6250000000000000000, 0.6500000000000000222, 0.6750000000000000444, 0.6999999999999999556, 0.7249999999999999778, 0.7500000000000000000, 0.7750000000000000222, 0.8000000000000000444, 0.8249999999999999556, 0.8499999999999999778, 0.8750000000000000000, 0.9000000000000000222, 0.9250000000000000444, 0.9499999999999999556, 0.9564318172069539159 ),
 .UNSPECIFIED. ) 
 CURVE ( )  GEOMETRIC_REPRESENTATION_ITEM ( )  RATIONAL_B_SPLINE_CURVE ( ( 1.000000000000000000, 0.9238795325112867385, 1.000000000000000000, 0.9238795325112867385, 1.000000000000000000, 0.9238795325112867385, 1.000000000000000000, 0.9238795325112867385, 1.000000000000000000, 0.9238795325112867385, 1.000000000000000000, 0.9238795325112867385, 1.000000000000000000, 0.9238795325112867385, 1.000000000000000000, 0.9238795325112867385, 1.000000000000000000, 0.9238795325112867385, 1.000000000000000000, 0.9238795325112867385, 1.000000000000000000, 0.9238795325112867385, 1.000000000000000000, 0.9238795325112867385, 1.000000000000000000, 0.9238795325112867385, 1.000000000000000000, 0.9238795325112867385, 1.000000000000000000, 0.9238795325112867385, 1.000000000000000000, 0.9238795325112867385, 1.000000000000000000, 0.9238795325112867385, 1.000000000000000000, 0.9238795325112867385, 1.000000000000000000, 0.9238795325112867385, 1.000000000000000000, 0.9238795325112867385, 1.000000000000000000, 0.9238795325112867385, 1.000000000000000000, 0.9238795325112867385, 1.000000000000000000, 0.9238795325112867385, 1.000000000000000000, 0.9238795325112867385, 1.000000000000000000, 0.9238795325112867385, 1.000000000000000000, 0.9238795325112867385, 1.000000000000000000, 0.9238795325112867385, 1.000000000000000000, 0.9238795325112867385, 1.000000000000000000, 0.9238795325112867385, 1.000000000000000000, 0.9238795325112867385, 1.000000000000000000, 0.9238795325112867385, 1.000000000000000000, 0.9238795325112867385, 1.000000000000000000, 0.9238795325112867385, 1.000000000000000000, 0.9238795325112867385, 1.000000000000000000, 0.9238795325112867385, 1.000000000000000000, 0.9238795325112867385, 1.000000000000000000, 0.9238795325112867385, 1.000000000000000000, 0.9238795325112867385, 1.000000000000000000, 0.9804162826961886346, 0.9709092765868392316 ) ) 
 REPRESENTATION_ITEM ( '' )  );
#4454=CARTESIAN_POINT ( 'NONE',  ( 10.19839929293505953, 3.581249999044085364, -24.62111388750000174 ) ) ;
#4464=CARTESIAN_POINT ( 'NONE',  ( 17.40975659021752620, 5.093749999044084653, 17.40975659021753330 ) ) ;
#4469=ORIENTED_EDGE ( 'NONE', *, *, #8601, .F. ) ;
#4475=DIRECTION ( 'NONE',  ( 0.000000000000000000, 0.000000000000000000, -1.000000000000000000 ) ) ;
#4477=DIRECTION ( 'NONE',  ( 0.000000000000000000, 0.000000000000000000, -1.000000000000000000 ) ) ;
#4485=ORIENTED_EDGE ( 'NONE', *, *, #256, .F. ) ;
#4489=CARTESIAN_POINT ( 'NONE',  ( 17.67766952966368521, 2.875000000000000000, 17.67766952966369232 ) ) ;
#4491=CARTESIAN_POINT ( 'NONE',  ( -4.522825247065398226E-15, 4.143749999044083587, 24.62111388750000174 ) ) ;
#4495=CIRCLE ( 'NONE', #8712, 24.91176187412963117 ) ;
#4506=DIRECTION ( 'NONE',  ( 0.000000000000000000, 0.000000000000000000, -1.000000000000000000 ) ) ;
#4507=ORIENTED_EDGE ( 'NONE', *, *, #8133, .F. ) ;
#4512=CARTESIAN_POINT ( 'NONE',  ( -17.67766952966368876, 0.9874999980881691286, -17.67766952966369232 ) ) ;
#4517=CARTESIAN_POINT ( 'NONE',  ( 17.40975659021752975, 3.343749999044085097, -17.40975659021752975 ) ) ;
#4522=( BOUNDED_CURVE ( )  B_SPLINE_CURVE ( 2, ( #5742, #8995, #9101, #1423, #4917, #3867, #8265, #5530, #1328 ),
 .UNSPECIFIED., .F., .F. ) 
 B_SPLINE_CURVE_WITH_KNOTS ( ( 3, 2, 2, 2, 3 ),
 ( 0.3499999999999999778, 0.3750000000000000000, 0.4000000000000000222, 0.4249999999999999889, 0.4500000000000000111 ),
 .UNSPECIFIED. ) 
 CURVE ( )  GEOMETRIC_REPRESENTATION_ITEM ( )  RATIONAL_B_SPLINE_CURVE ( ( 1.000000000000000000, 0.9238795325112867385, 1.000000000000000000, 0.9238795325112867385, 1.000000000000000000, 0.9238795325112867385, 1.000000000000000000, 0.9238795325112867385, 1.000000000000000000 ) ) 
 REPRESENTATION_ITEM ( '' )  );
#4525=DIRECTION ( 'NONE',  ( 1.000000000000000000, 0.000000000000000000, -0.000000000000000000 ) ) ;
#4546=CARTESIAN_POINT ( 'NONE',  ( 10.19839929293506486, 3.206249999044084031, 24.62111388749999819 ) ) ;
#4553=CARTESIAN_POINT ( 'NONE',  ( -23.92316786293533681, 5.000000000000000000, 6.437029362807039412 ) ) ;
#4559=CARTESIAN_POINT ( 'NONE',  ( -24.62111388750000174, 4.656249999044085541, -10.19839929293506131 ) ) ;
#4566=CARTESIAN_POINT ( 'NONE',  ( 24.62111388749999463, 1.156249999044084431, 10.19839929293507730 ) ) ;
#4567=CONICAL_SURFACE ( 'NONE', #2580, 25.00000000000000000, 0.3490658503988666728 ) ;
#4579=EDGE_CURVE ( 'NONE', #7487, #2886, #6297, .T. ) ;
#4595=CARTESIAN_POINT ( 'NONE',  ( 24.62111388750000174, 3.393749999044084475, 0.000000000000000000 ) ) ;
#4602=EDGE_CURVE ( 'NONE', #2139, #3676, #8000, .T. ) ;
#4611=CARTESIAN_POINT ( 'NONE',  ( 17.40975659021752620, 2.093749999044084653, 17.40975659021753330 ) ) ;
#4618=CARTESIAN_POINT ( 'NONE',  ( -4.522825247065398226E-15, 3.968749999044084209, 24.62111388750000174 ) ) ;
#4625=CARTESIAN_POINT ( 'NONE',  ( 0.000000000000000000, 5.000000000000000000, 0.000000000000000000 ) ) ;
#4644=EDGE_CURVE ( 'NONE', #292, #39, #9656, .T. ) ;
#4651=ADVANCED_FACE ( 'NONE', ( #4901 ), #5376, .T. ) ;
#4660=ADVANCED_FACE ( 'NONE', ( #9804 ), #9041, .F. ) ;
#4665=CARTESIAN_POINT ( 'NONE',  ( -4.522825247065398226E-15, 4.968749999044083765, 24.62111388750000174 ) ) ;
#4674=CARTESIAN_POINT ( 'NONE',  ( -10.19839929293505776, 3.531249999044084653, -24.62111388750000174 ) ) ;
#4683=CARTESIAN_POINT ( 'NONE',  ( 10.35533905932737930, 2.187500000000000444, -25.00000000000000000 ) ) ;
#4687=ORIENTED_EDGE ( 'NONE', *, *, #4579, .T. ) ;
#4692=FACE_OUTER_BOUND ( 'NONE', #10534, .T. ) ;
#4711=CARTESIAN_POINT ( 'NONE',  ( 4.895565917430008795, 5.000000000000001776, 24.12949820052922334 ) ) ;
#4712=CARTESIAN_POINT ( 'NONE',  ( 1.530808498934191521E-15, 4.250000000000000000, -25.00000000000000000 ) ) ;
#4717=CARTESIAN_POINT ( 'NONE',  ( -24.62111388750000174, 2.718749999044084653, -3.015216831376932151E-15 ) ) ;
#4726=CARTESIAN_POINT ( 'NONE',  ( -25.00000000000001421, 2.562500000000000444, 10.35533905932737397 ) ) ;
#4729=ORIENTED_EDGE ( 'NONE', *, *, #10313, .F. ) ;
#4730=ADVANCED_FACE ( 'NONE', ( #3002 ), #9088, .T. ) ;
#4743=EDGE_CURVE ( 'NONE', #10892, #8014, #589, .T. ) ;
#4760=CARTESIAN_POINT ( 'NONE',  ( -24.62111388750000174, 2.718749999044084653, -3.015216831376932151E-15 ) ) ;
#4764=VERTEX_POINT ( 'NONE', #9972 ) ;
#4766=CARTESIAN_POINT ( 'NONE',  ( 17.67766952966368521, 3.487499998088169129, 17.67766952966369232 ) ) ;
#4785=COLOUR_RGB ( '', 0.09019608, 0.27058824, 0.51372549) ;
#4788=EDGE_CURVE ( 'NONE', #10138, #6596, #1746, .T. ) ;
#4800=DIRECTION ( 'NONE',  ( 0.000000000000000000, 0.000000000000000000, 1.000000000000000000 ) ) ;
#4815=CARTESIAN_POINT ( 'NONE',  ( 1.530808498934191521E-15, 1.250000000000000000, -25.00000000000000000 ) ) ;
#4821=AXIS2_PLACEMENT_3D ( 'NONE', #5297, #1097, #4475 ) ;
#4822=ORIENTED_EDGE ( 'NONE', *, *, #2585, .F. ) ;
#4823=CARTESIAN_POINT ( 'NONE',  ( 10.35533905932738286, 3.424999998088169573, 24.99999999999999645 ) ) ;
#4825=AXIS2_PLACEMENT_3D ( 'NONE', #10074, #5940, #5888 ) ;
#4849=CARTESIAN_POINT ( 'NONE',  ( -10.19839929293507552, 1.906249999044084431, 24.62111388749999463 ) ) ;
#4850=FACE_OUTER_BOUND ( 'NONE', #3079, .T. ) ;
#4854=EDGE_LOOP ( 'NONE', ( #9018, #1910, #6041, #9478 ) ) ;
#4856=CARTESIAN_POINT ( 'NONE',  ( 0.000000000000000000, 0.000000000000000000, 0.000000000000000000 ) ) ;
#4857=EDGE_CURVE ( 'NONE', #9230, #1424, #10917, .T. ) ;
#4875=CARTESIAN_POINT ( 'NONE',  ( 25.00000000000000000, 4.612499998088169129, 0.000000000000000000 ) ) ;
#4888=CARTESIAN_POINT ( 'NONE',  ( -17.99166497301935408, 4.999999999999999112, 16.96057692830995478 ) ) ;
#4891=CARTESIAN_POINT ( 'NONE',  ( -24.62111388750000174, 1.656249999044084431, -10.19839929293506131 ) ) ;
#4901=FACE_OUTER_BOUND ( 'NONE', #3999, .T. ) ;
#4904=CARTESIAN_POINT ( 'NONE',  ( 25.00000000000000000, 1.000000000000000000, 0.000000000000000000 ) ) ;
#4914=ORIENTED_EDGE ( 'NONE', *, *, #9276, .F. ) ;
#4917=CARTESIAN_POINT ( 'NONE',  ( 25.00000000000000000, 2.612499998088169129, 0.000000000000000000 ) ) ;
#4925=ORIENTED_EDGE ( 'NONE', *, *, #6294, .F. ) ;
#4926=EDGE_CURVE ( 'NONE', #3614, #69, #8347, .T. ) ;
#4927=CARTESIAN_POINT ( 'NONE',  ( 17.67766952966369232, 2.737499998088169573, -17.67766952966369232 ) ) ;
#4944=CARTESIAN_POINT ( 'NONE',  ( 0.000000000000000000, -1.026060429977008193, 0.000000000000000000 ) ) ;
#4945=CARTESIAN_POINT ( 'NONE',  ( 0.000000000000000000, -8.528980942125404141, -24.91176187412963117 ) ) ;
#4972=ORIENTED_EDGE ( 'NONE', *, *, #3989, .F. ) ;
#4981=EDGE_LOOP ( 'NONE', ( #9024, #286, #2983, #8297 ) ) ;
#4983=CARTESIAN_POINT ( 'NONE',  ( -10.19839929293507552, 1.081249999044084475, 24.62111388749999463 ) ) ;
#5004=CARTESIAN_POINT ( 'NONE',  ( 25.00000000000000000, 3.062500000000000000, -10.35533905932737753 ) ) ;
#5006=CIRCLE ( 'NONE', #240, 24.91176187412963117 ) ;
#5008=CARTESIAN_POINT ( 'NONE',  ( -25.00000000000000000, 2.112499998088169129, -3.061616997868383043E-15 ) ) ;
#5012=CARTESIAN_POINT ( 'NONE',  ( 24.62111388750000174, 2.218749999044084653, 0.000000000000000000 ) ) ;
#5019=CIRCLE ( 'NONE', #9606, 27.91176187412962761 ) ;
#5031=ORIENTED_EDGE ( 'NONE', *, *, #8067, .F. ) ;
#5058=CARTESIAN_POINT ( 'NONE',  ( 17.40975659021752975, 0.3437499990440845421, -17.40975659021752975 ) ) ;
#5064=CARTESIAN_POINT ( 'NONE',  ( 24.62111388750000174, 2.281249999044085541, -10.19839929293505776 ) ) ;
#5074=CARTESIAN_POINT ( 'NONE',  ( 24.99999999999999289, 4.937500000000000888, 10.35533905932739529 ) ) ;
#5075=ADVANCED_BREP_SHAPE_REPRESENTATION ( '', ( #3340, #7040 ), #8059 ) ;
#5090=CARTESIAN_POINT ( 'NONE',  ( -4.592425496802574367E-15, 1.362499998088169129, 25.00000000000000000 ) ) ;
#5096=CARTESIAN_POINT ( 'NONE',  ( 17.67766952966369232, 1.737499998088169351, -17.67766952966369232 ) ) ;
#5103=CARTESIAN_POINT ( 'NONE',  ( 1.507608415688466075E-15, 3.643749999044084920, -24.62111388750000174 ) ) ;
#5108=ORIENTED_EDGE ( 'NONE', *, *, #5539, .T. ) ;
#5109=CARTESIAN_POINT ( 'NONE',  ( -17.67766952966369232, 2.237499998088169573, 17.67766952966368876 ) ) ;
#5111=CARTESIAN_POINT ( 'NONE',  ( 24.99999999999999289, 0.9374999999999998890, 10.35533905932739529 ) ) ;
#5115=VERTEX_POINT ( 'NONE', #2285 ) ;
#5118=CARTESIAN_POINT ( 'NONE',  ( 2.694222958124177204E-15, 5.000000000000000000, 22.00000000000000355 ) ) ;
#5137=CARTESIAN_POINT ( 'NONE',  ( -25.00000000000000000, 4.437500000000001776, -10.35533905932738108 ) ) ;
#5140=DIRECTION ( 'NONE',  ( 0.000000000000000000, -1.000000000000000000, 0.000000000000000000 ) ) ;
#5149=CARTESIAN_POINT ( 'NONE',  ( 24.62111388750000174, 1.456249999044084475, -10.19839929293505776 ) ) ;
#5157=CARTESIAN_POINT ( 'NONE',  ( 1.530808498934191521E-15, 1.862499998088169129, -25.00000000000000000 ) ) ;
#5159=CARTESIAN_POINT ( 'NONE',  ( -4.592425496802574367E-15, 3.750000000000000000, 25.00000000000000000 ) ) ;
#5160=CIRCLE ( 'NONE', #9728, 24.91176187412963117 ) ;
#5167=CARTESIAN_POINT ( 'NONE',  ( -24.62111388750000174, 2.831249999044084475, -10.19839929293506131 ) ) ;
#5168=CIRCLE ( 'NONE', #3919, 25.00000000000000000 ) ;
#5175=DIRECTION ( 'NONE',  ( 0.000000000000000000, 0.000000000000000000, -1.000000000000000000 ) ) ;
#5177=CARTESIAN_POINT ( 'NONE',  ( -17.40975659021752975, 4.593749999044084653, -17.40975659021752975 ) ) ;
#5178=CARTESIAN_POINT ( 'NONE',  ( -25.00000000000000000, 3.049999998088169129, -10.35533905932738108 ) ) ;
#5189=EDGE_CURVE ( 'NONE', #10065, #9967, #7211, .T. ) ;
#5197=CARTESIAN_POINT ( 'NONE',  ( 20.15540488255180307, 5.000000000000000000, 14.56419990634798900 ) ) ;
#5199=ADVANCED_FACE ( 'NONE', ( #10737 ), #3899, .T. ) ;
#5203=AXIS2_PLACEMENT_3D ( 'NONE', #5622, #7428, #7317 ) ;
#5207=CARTESIAN_POINT ( 'NONE',  ( -10.19839929293507375, 2.081249999044084920, 24.62111388749999108 ) ) ;
#5213=CARTESIAN_POINT ( 'NONE',  ( -24.62111388750000884, 3.956249999044084920, 10.19839929293505421 ) ) ;
#5219=PRESENTATION_STYLE_ASSIGNMENT (( #4441 ) ) ;
#5221=CARTESIAN_POINT ( 'NONE',  ( 24.62111388750000174, 0.2812499990440845421, -10.19839929293505776 ) ) ;
#5224=CARTESIAN_POINT ( 'NONE',  ( 17.67766952966368521, 3.875000000000000000, 17.67766952966369232 ) ) ;
#5229=CARTESIAN_POINT ( 'NONE',  ( -10.19839929293507552, 4.081249999044084475, 24.62111388749999463 ) ) ;
#5238=CARTESIAN_POINT ( 'NONE',  ( 10.35533905932738286, 0.8125000000000001110, 24.99999999999999645 ) ) ;
#5246=DIRECTION ( 'NONE',  ( 0.000000000000000000, -1.000000000000000000, 0.000000000000000000 ) ) ;
#5255=CARTESIAN_POINT ( 'NONE',  ( -10.19839929293505776, 1.706249999044084698, -24.62111388750000174 ) ) ;
#5270=DIRECTION ( 'NONE',  ( 0.000000000000000000, -1.000000000000000000, 0.000000000000000000 ) ) ;
#5271=VECTOR ( 'NONE', #10476, 999.9999999999998863 ) ;
#5274=CARTESIAN_POINT ( 'NONE',  ( 24.99999999999999289, 2.937500000000000444, 10.35533905932739529 ) ) ;
#5277=ORIENTED_EDGE ( 'NONE', *, *, #8492, .F. ) ;
#5281=CARTESIAN_POINT ( 'NONE',  ( -4.522825247065398226E-15, 4.143749999044084475, 24.62111388750000174 ) ) ;
#5292=CARTESIAN_POINT ( 'NONE',  ( 24.62111388750000174, 4.281249999044084653, -10.19839929293505776 ) ) ;
#5297=CARTESIAN_POINT ( 'NONE',  ( 0.000000000000000000, 5.000000000000000000, 0.000000000000000000 ) ) ;
#5301=DIRECTION ( 'NONE',  ( 0.000000000000000000, -1.000000000000000000, 0.000000000000000000 ) ) ;
#5310=CARTESIAN_POINT ( 'NONE',  ( -24.62111388750000884, 2.956249999044084475, 10.19839929293505421 ) ) ;
#5318=AXIS2_PLACEMENT_3D ( 'NONE', #6217, #2918, #2969 ) ;
#5323=VERTEX_POINT ( 'NONE', #4381 ) ;
#5325=EDGE_CURVE ( 'NONE', #10743, #2663, #4448, .T. ) ;
#5328=CARTESIAN_POINT ( 'NONE',  ( -17.67766952966369232, 1.237499998088169129, 17.67766952966368876 ) ) ;
#5331=ORIENTED_EDGE ( 'NONE', *, *, #10318, .F. ) ;
#5334=CARTESIAN_POINT ( 'NONE',  ( -17.40975659021753330, 1.843749999044084653, 17.40975659021752975 ) ) ;
#5343=CARTESIAN_POINT ( 'NONE',  ( -10.35533905932739174, 1.687500000000000000, 24.99999999999999289 ) ) ;
#5346=ORIENTED_EDGE ( 'NONE', *, *, #6071, .T. ) ;
#5351=VECTOR ( 'NONE', #8677, 1000.000000000000000 ) ;
#5367=CARTESIAN_POINT ( 'NONE',  ( -4.592425496802574367E-15, 1.362499998088169129, 25.00000000000000000 ) ) ;
#5368=CARTESIAN_POINT ( 'NONE',  ( -24.62111388750000174, 2.831249999044084475, -10.19839929293506131 ) ) ;
#5373=DIRECTION ( 'NONE',  ( 0.000000000000000000, 0.000000000000000000, -1.000000000000000000 ) ) ;
#5376=CONICAL_SURFACE ( 'NONE', #6076, 25.00000000000000000, 0.3490658503988666728 ) ;
#5382=VERTEX_POINT ( 'NONE', #6687 ) ;
#5385=CARTESIAN_POINT ( 'NONE',  ( -4.522825247065398226E-15, 2.968749999044084653, 24.62111388750000174 ) ) ;
#5391=CARTESIAN_POINT ( 'NONE',  ( 10.19839929293506486, 1.031249999044084653, 24.62111388749999819 ) ) ;
#5396=EDGE_CURVE ( 'NONE', #6575, #9230, #7520, .T. ) ;
#5400=DIRECTION ( 'NONE',  ( 0.000000000000000000, -1.000000000000000000, 0.000000000000000000 ) ) ;
#5403=ORIENTED_EDGE ( 'NONE', *, *, #8009, .T. ) ;
#5407=CYLINDRICAL_SURFACE ( 'NONE', #4821, 22.00000000000000355 ) ;
#5411=CARTESIAN_POINT ( 'NONE',  ( 24.62111388750000174, 0.2812499990440845976, -10.19839929293505776 ) ) ;
#5415=CARTESIAN_POINT ( 'NONE',  ( -24.62111388750000884, 3.956249999044084475, 10.19839929293505421 ) ) ;
#5420=ORIENTED_EDGE ( 'NONE', *, *, #4788, .T. ) ;
#5425=ORIENTED_EDGE ( 'NONE', *, *, #8734, .T. ) ;
#5428=CARTESIAN_POINT ( 'NONE',  ( -10.19839929293507375, 1.906249999044084431, 24.62111388749999108 ) ) ;
#5433=CARTESIAN_POINT ( 'NONE',  ( 24.62111388750000174, 3.218749999044084653, 0.000000000000000000 ) ) ;
#5441=CARTESIAN_POINT ( 'NONE',  ( 0.000000000000000000, 5.000000000000000000, 0.000000000000000000 ) ) ;
#5447=CARTESIAN_POINT ( 'NONE',  ( 25.00000000000000000, 0.6124999980881691286, 0.000000000000000000 ) ) ;
#5476=CARTESIAN_POINT ( 'NONE',  ( -10.19839929293507375, 4.906249999044083765, 24.62111388749999108 ) ) ;
#5480=CIRCLE ( 'NONE', #5656, 25.00000000000000000 ) ;
#5483=CARTESIAN_POINT ( 'NONE',  ( 24.62111388749999463, 4.156249999044083765, 10.19839929293507730 ) ) ;
#5495=ORIENTED_EDGE ( 'NONE', *, *, #5189, .T. ) ;
#5503=CARTESIAN_POINT ( 'NONE',  ( 0.000000000000000000, 5.000000000000000000, 0.000000000000000000 ) ) ;
#5510=CARTESIAN_POINT ( 'NONE',  ( 0.000000000000000000, 5.000000000000000000, 0.000000000000000000 ) ) ;
#5520=ORIENTED_EDGE ( 'NONE', *, *, #388, .F. ) ;
#5530=CARTESIAN_POINT ( 'NONE',  ( 10.35533905932737930, 2.799999998088169573, -25.00000000000000000 ) ) ;
#5533=CARTESIAN_POINT ( 'NONE',  ( 24.62111388749999108, 3.156249999044084653, 10.19839929293507730 ) ) ;
#5534=CARTESIAN_POINT ( 'NONE',  ( 0.000000000000000000, 0.000000000000000000, 0.000000000000000000 ) ) ;
#5539=EDGE_CURVE ( 'NONE', #1367, #4397, #7610, .T. ) ;
#5541=CIRCLE ( 'NONE', #9228, 25.00000000000000000 ) ;
#5543=CARTESIAN_POINT ( 'NONE',  ( -4.522825247065398226E-15, 2.968749999044084653, 24.62111388750000174 ) ) ;
#5552=EDGE_CURVE ( 'NONE', #2139, #292, #6798, .T. ) ;
#5564=( BOUNDED_CURVE ( )  B_SPLINE_CURVE ( 2, ( #1415, #9091, #5733, #2450, #4904, #3061, #10651, #1520, #4021 ),
 .UNSPECIFIED., .F., .F. ) 
 B_SPLINE_CURVE_WITH_KNOTS ( ( 3, 2, 2, 2, 3 ),
 ( 0.1500000000000000222, 0.1750000000000000167, 0.2000000000000000389, 0.2250000000000000333, 0.2500000000000000000 ),
 .UNSPECIFIED. ) 
 CURVE ( )  GEOMETRIC_REPRESENTATION_ITEM ( )  RATIONAL_B_SPLINE_CURVE ( ( 0.9999999999999998890, 0.9238795325112868495, 1.000000000000000000, 0.9238795325112867385, 1.000000000000000000, 0.9238795325112867385, 1.000000000000000000, 0.9238795325112867385, 1.000000000000000000 ) ) 
 REPRESENTATION_ITEM ( '' )  );
#5567=EDGE_LOOP ( 'NONE', ( #7417, #1632, #1993, #7883 ) ) ;
#5569=CARTESIAN_POINT ( 'NONE',  ( 25.00000000000000000, 0.6749999980881691286, -10.35533905932737753 ) ) ;
#5584=CARTESIAN_POINT ( 'NONE',  ( 24.62111388750000174, 3.281249999044084653, -10.19839929293505776 ) ) ;
#5591=CARTESIAN_POINT ( 'NONE',  ( 17.40975659021752975, 0.5187499990440845865, -17.40975659021752975 ) ) ;
#5602=EDGE_LOOP ( 'NONE', ( #7158, #7068, #10231, #2260 ) ) ;
#5622=CARTESIAN_POINT ( 'NONE',  ( 0.000000000000000000, 5.000000000000000000, 0.000000000000000000 ) ) ;
#5624=( BOUNDED_CURVE ( )  B_SPLINE_CURVE ( 2, ( #1148, #1795, #7927, #7053, #10408, #2826, #6225, #6827, #9587 ),
 .UNSPECIFIED., .F., .F. ) 
 B_SPLINE_CURVE_WITH_KNOTS ( ( 3, 2, 2, 2, 3 ),
 ( 0.4500000000000000111, 0.4749999999999999778, 0.5000000000000000000, 0.5250000000000000222, 0.5500000000000000444 ),
 .UNSPECIFIED. ) 
 CURVE ( )  GEOMETRIC_REPRESENTATION_ITEM ( )  RATIONAL_B_SPLINE_CURVE ( ( 1.000000000000000000, 0.9238795325112867385, 1.000000000000000000, 0.9238795325112867385, 1.000000000000000000, 0.9238795325112867385, 1.000000000000000000, 0.9238795325112867385, 1.000000000000000000 ) ) 
 REPRESENTATION_ITEM ( '' )  );
#5635=CARTESIAN_POINT ( 'NONE',  ( 25.00000000000000000, 3.674999998088170017, -10.35533905932737753 ) ) ;
#5646=CARTESIAN_POINT ( 'NONE',  ( -25.00000000000000000, 4.112499998088169129, -3.061616997868383043E-15 ) ) ;
#5656=AXIS2_PLACEMENT_3D ( 'NONE', #1543, #2316, #4043 ) ;
#5661=EDGE_CURVE ( 'NONE', #10861, #9966, #4495, .T. ) ;
#5664=DIRECTION ( 'NONE',  ( 0.000000000000000000, -1.000000000000000000, 0.000000000000000000 ) ) ;
#5668=CARTESIAN_POINT ( 'NONE',  ( 10.19839929293506486, 4.031249999044083765, 24.62111388749999819 ) ) ;
#5669=DIRECTION ( 'NONE',  ( 0.000000000000000000, 0.000000000000000000, -1.000000000000000000 ) ) ;
#5692=CARTESIAN_POINT ( 'NONE',  ( -17.67766952966368876, 1.375000000000000000, -17.67766952966369232 ) ) ;
#5699=CARTESIAN_POINT ( 'NONE',  ( -24.62111388750000174, 0.8937499990440845865, -3.015216831376932151E-15 ) ) ;
#5706=DIRECTION ( 'NONE',  ( 0.000000000000000000, 0.000000000000000000, -1.000000000000000000 ) ) ;
#5712=EDGE_CURVE ( 'NONE', #9230, #6463, #2136, .T. ) ;
#5715=UNCERTAINTY_MEASURE_WITH_UNIT (LENGTH_MEASURE( 1.000000000000000082E-05 ), #1890, 'distance_accuracy_value', 'NONE');
#5722=CARTESIAN_POINT ( 'NONE',  ( -4.522825247065398226E-15, 2.968749999044084653, 24.62111388750000174 ) ) ;
#5723=CARTESIAN_POINT ( 'NONE',  ( 2.716379529800028356E-15, -1.026060429977008193, 22.18092213764227694 ) ) ;
#5733=CARTESIAN_POINT ( 'NONE',  ( 17.67766952966368521, 0.8750000000000000000, 17.67766952966369232 ) ) ;
#5737=PRESENTATION_STYLE_ASSIGNMENT (( #2359 ) ) ;
#5741=CARTESIAN_POINT ( 'NONE',  ( 10.35533905932738286, 3.424999998088169129, 24.99999999999999645 ) ) ;
#5742=CARTESIAN_POINT ( 'NONE',  ( -4.592425496802574367E-15, 2.362499998088169129, 25.00000000000000000 ) ) ;
#5746=CARTESIAN_POINT ( 'NONE',  ( -10.35533905932737575, 2.924999998088168685, -25.00000000000000000 ) ) ;
#5756=APPLICATION_CONTEXT ( 'automotive_design' ) ;
#5759=DIRECTION ( 'NONE',  ( 0.000000000000000000, 0.000000000000000000, -1.000000000000000000 ) ) ;
#5763=CARTESIAN_POINT ( 'NONE',  ( -24.62111388750000884, 0.7812499990440845421, 10.19839929293505421 ) ) ;
#5765=CARTESIAN_POINT ( 'NONE',  ( 10.19839929293506486, 2.031249999044084653, 24.62111388749999819 ) ) ;
#5768=EDGE_CURVE ( 'NONE', #4764, #6575, #5564, .T. ) ;
#5781=CARTESIAN_POINT ( 'NONE',  ( 14.02827699982873888, 5.000000000000000888, 20.42037923990229942 ) ) ;
#5800=CARTESIAN_POINT ( 'NONE',  ( -17.40975659021753330, 1.018749999044084698, 17.40975659021752975 ) ) ;
#5801=CARTESIAN_POINT ( 'NONE',  ( 1.530808498934191521E-15, 3.862499998088169573, -25.00000000000000000 ) ) ;
#5815=FACE_OUTER_BOUND ( 'NONE', #5602, .T. ) ;
#5823=CARTESIAN_POINT ( 'NONE',  ( -17.40975659021753330, 0.8437499990440846531, 17.40975659021752975 ) ) ;
#5826=ORIENTED_EDGE ( 'NONE', *, *, #5189, .F. ) ;
#5838=VERTEX_POINT ( 'NONE', #9144 ) ;
#5839=( BOUNDED_CURVE ( )  B_SPLINE_CURVE ( 2, ( #5367, #274, #7307, #8726, #1168, #1108, #1399, #10735, #10630 ),
 .UNSPECIFIED., .F., .F. ) 
 B_SPLINE_CURVE_WITH_KNOTS ( ( 3, 2, 2, 2, 3 ),
 ( 0.1499999999999999944, 0.1749999999999999889, 0.2000000000000000111, 0.2249999999999999778, 0.2499999999999999722 ),
 .UNSPECIFIED. ) 
 CURVE ( )  GEOMETRIC_REPRESENTATION_ITEM ( )  RATIONAL_B_SPLINE_CURVE ( ( 1.000000000000000000, 0.9238795325112867385, 1.000000000000000000, 0.9238795325112867385, 1.000000000000000000, 0.9238795325112867385, 1.000000000000000000, 0.9238795325112868495, 0.9999999999999998890 ) ) 
 REPRESENTATION_ITEM ( '' )  );
#5858=CARTESIAN_POINT ( 'NONE',  ( -24.62111388750000174, 3.831249999044084920, -10.19839929293506131 ) ) ;
#5883=CARTESIAN_POINT ( 'NONE',  ( -19.39162934935757931, 5.000000000000000888, 15.17115553405142947 ) ) ;
#5884=CARTESIAN_POINT ( 'NONE',  ( -4.592425496802574367E-15, 4.362499998088169129, 25.00000000000000000 ) ) ;
#5886=ADVANCED_FACE ( 'NONE', ( #90 ), #8539, .T. ) ;
#5887=CARTESIAN_POINT ( 'NONE',  ( 1.507608415688466075E-15, 3.468749999044085097, -24.62111388750000174 ) ) ;
#5888=DIRECTION ( 'NONE',  ( 0.000000000000000000, 0.000000000000000000, -1.000000000000000000 ) ) ;
#5890=VERTEX_POINT ( 'NONE', #9305 ) ;
#5913=( BOUNDED_CURVE ( )  B_SPLINE_CURVE ( 2, ( #5884, #4219, #9238, #5938, #6655, #912, #4281, #10015, #2439 ),
 .UNSPECIFIED., .F., .F. ) 
 B_SPLINE_CURVE_WITH_KNOTS ( ( 3, 2, 2, 2, 3 ),
 ( 0.7500000000000000000, 0.7750000000000000222, 0.8000000000000000444, 0.8250000000000000666, 0.8500000000000000888 ),
 .UNSPECIFIED. ) 
 CURVE ( )  GEOMETRIC_REPRESENTATION_ITEM ( )  RATIONAL_B_SPLINE_CURVE ( ( 1.000000000000000000, 0.9238795325112867385, 1.000000000000000000, 0.9238795325112867385, 1.000000000000000000, 0.9238795325112867385, 1.000000000000000000, 0.9238795325112864054, 1.000000000000000444 ) ) 
 REPRESENTATION_ITEM ( '' )  );
#5915=CARTESIAN_POINT ( 'NONE',  ( -24.62111388750000174, 3.893749999044084475, -3.015216831376932151E-15 ) ) ;
#5917=DIRECTION ( 'NONE',  ( -0.000000000000000000, 1.000000000000000000, -0.000000000000000000 ) ) ;
#5923=CARTESIAN_POINT ( 'NONE',  ( 25.00000000000000000, 0.6124999980881691286, 0.000000000000000000 ) ) ;
#5931=ADVANCED_FACE ( 'NONE', ( #6073 ), #866, .F. ) ;
#5932=CARTESIAN_POINT ( 'NONE',  ( 24.62111388750000174, 3.456249999044084920, -10.19839929293505776 ) ) ;
#5938=CARTESIAN_POINT ( 'NONE',  ( 24.99999999999999289, 4.549999998088169129, 10.35533905932739529 ) ) ;
#5939=CARTESIAN_POINT ( 'NONE',  ( -10.35533905932737575, 0.3125000000000000000, -25.00000000000000000 ) ) ;
#5940=DIRECTION ( 'NONE',  ( 0.000000000000000000, -1.000000000000000000, 0.000000000000000000 ) ) ;
#5944=CARTESIAN_POINT ( 'NONE',  ( 1.530808498934191521E-15, 2.862499998088169573, -25.00000000000000000 ) ) ;
#5947=CARTESIAN_POINT ( 'NONE',  ( 25.00000000000000000, 2.000000000000000000, 0.000000000000000000 ) ) ;
#5969=CARTESIAN_POINT ( 'NONE',  ( 24.62111388750000174, 0.4562499990440845865, -10.19839929293505776 ) ) ;
#5970=CARTESIAN_POINT ( 'NONE',  ( -10.19839929293505776, 3.706249999044084920, -24.62111388750000174 ) ) ;
#5979=CARTESIAN_POINT ( 'NONE',  ( 25.00000000000000000, 1.612499998088169351, 0.000000000000000000 ) ) ;
#5988=CARTESIAN_POINT ( 'NONE',  ( -17.40975659021752975, 3.768749999044084475, -17.40975659021752975 ) ) ;
#5995=CARTESIAN_POINT ( 'NONE',  ( 2.668943309558227117, 5.000000000000000888, 24.58125138907406537 ) ) ;
#5997=CARTESIAN_POINT ( 'NONE',  ( -4.522825247065398226E-15, 4.968749999044083765, 24.62111388750000174 ) ) ;
#6005=CARTESIAN_POINT ( 'NONE',  ( -25.00000000000000000, 4.049999998088169129, -10.35533905932738108 ) ) ;
#6020=CARTESIAN_POINT ( 'NONE',  ( -17.67766952966369232, 4.625000000000000000, 17.67766952966368876 ) ) ;
#6022=CARTESIAN_POINT ( 'NONE',  ( 24.62111388750000174, 4.393749999044084475, 0.000000000000000000 ) ) ;
#6028=CARTESIAN_POINT ( 'NONE',  ( 24.62111388750000174, 1.456249999044084475, -10.19839929293505776 ) ) ;
#6029=CARTESIAN_POINT ( 'NONE',  ( -24.62111388750000174, 1.893749999044084475, -3.015216831376932151E-15 ) ) ;
#6034=CARTESIAN_POINT ( 'NONE',  ( 0.000000000000000000, 5.000000000000000000, 0.000000000000000000 ) ) ;
#6037=CARTESIAN_POINT ( 'NONE',  ( 24.99999999999999289, 2.549999998088169129, 10.35533905932739529 ) ) ;
#6039=CARTESIAN_POINT ( 'NONE',  ( -10.35533905932739174, 2.687500000000000888, 24.99999999999999289 ) ) ;
#6041=ORIENTED_EDGE ( 'NONE', *, *, #8492, .T. ) ;
#6046=CARTESIAN_POINT ( 'NONE',  ( 1.507608415688466075E-15, 2.643749999044084920, -24.62111388750000174 ) ) ;
#6071=EDGE_CURVE ( 'NONE', #8219, #1642, #5006, .T. ) ;
#6073=FACE_OUTER_BOUND ( 'NONE', #7997, .T. ) ;
#6076=AXIS2_PLACEMENT_3D ( 'NONE', #4856, #6405, #7371 ) ;
#6085=CARTESIAN_POINT ( 'NONE',  ( 10.19839929293506486, 2.206249999044084920, 24.62111388749999819 ) ) ;
#6089=DIRECTION ( 'NONE',  ( 0.000000000000000000, 1.000000000000000000, 0.000000000000000000 ) ) ;
#6091=CARTESIAN_POINT ( 'NONE',  ( 10.19839929293505953, 1.581249999044084475, -24.62111388750000174 ) ) ;
#6092=CARTESIAN_POINT ( 'NONE',  ( -17.40975659021753330, 4.018749999044084475, 17.40975659021752975 ) ) ;
#6098=( NAMED_UNIT ( * ) SI_UNIT ( $, .STERADIAN. ) SOLID_ANGLE_UNIT ( ) );
#6101=CARTESIAN_POINT ( 'NONE',  ( -25.00000000000000000, 1.112499998088169351, -3.061616997868383043E-15 ) ) ;
#6103=CARTESIAN_POINT ( 'NONE',  ( -25.00000000000000000, 3.437500000000000000, -10.35533905932738108 ) ) ;
#6107=CARTESIAN_POINT ( 'NONE',  ( -10.19839929293505776, 3.706249999044084920, -24.62111388750000174 ) ) ;
#6124=CARTESIAN_POINT ( 'NONE',  ( 3.050810944027392283E-15, -55.00000000000000000, -24.91176187412963117 ) ) ;
#6133=CARTESIAN_POINT ( 'NONE',  ( 17.40975659021752620, 3.268749999044084475, 17.40975659021753330 ) ) ;
#6134=CARTESIAN_POINT ( 'NONE',  ( 0.000000000000000000, 0.000000000000000000, 0.000000000000000000 ) ) ;
#6151=CARTESIAN_POINT ( 'NONE',  ( 10.35533905932737930, 0.7999999980881692396, -25.00000000000000000 ) ) ;
#6156=CARTESIAN_POINT ( 'NONE',  ( -10.19839929293507552, 2.081249999044084475, 24.62111388749999463 ) ) ;
#6158=VECTOR ( 'NONE', #1295, 1000.000000000000000 ) ;
#6159=FACE_OUTER_BOUND ( 'NONE', #3871, .T. ) ;
#6160=CARTESIAN_POINT ( 'NONE',  ( 24.62111388750000174, 5.393749999044085364, 0.000000000000000000 ) ) ;
#6170=CARTESIAN_POINT ( 'NONE',  ( -17.67766952966368876, 0.3750000000000000000, -17.67766952966369232 ) ) ;
#6190=CARTESIAN_POINT ( 'NONE',  ( -17.40975659021752975, 1.768749999044084475, -17.40975659021752975 ) ) ;
#6195=CIRCLE ( 'NONE', #1406, 2.999999999999999112 ) ;
#6198=EDGE_LOOP ( 'NONE', ( #7750, #5520, #8635 ) ) ;
#6209=CARTESIAN_POINT ( 'NONE',  ( -24.62111388750000174, 1.656249999044084431, -10.19839929293506131 ) ) ;
#6217=CARTESIAN_POINT ( 'NONE',  ( 0.000000000000000000, -58.00000000000000000, 0.000000000000000000 ) ) ;
#6218=CARTESIAN_POINT ( 'NONE',  ( -10.19839929293507552, 1.906249999044084431, 24.62111388749999463 ) ) ;
#6225=CARTESIAN_POINT ( 'NONE',  ( -17.67766952966369232, 2.625000000000000000, 17.67766952966368876 ) ) ;
#6228=CARTESIAN_POINT ( 'NONE',  ( 24.99999999999999289, 1.937500000000000000, 10.35533905932739529 ) ) ;
#6249=CARTESIAN_POINT ( 'NONE',  ( 24.62111388750000174, 2.393749999044084475, 0.000000000000000000 ) ) ;
#6260=ORIENTED_EDGE ( 'NONE', *, *, #9519, .F. ) ;
#6264=CARTESIAN_POINT ( 'NONE',  ( -10.19839929293505776, 3.531249999044084653, -24.62111388750000174 ) ) ;
#6273=CARTESIAN_POINT ( 'NONE',  ( 24.62111388749999463, 3.156249999044084653, 10.19839929293507730 ) ) ;
#6277=CARTESIAN_POINT ( 'NONE',  ( 0.000000000000000000, 5.000000000000000000, -25.00000000000000000 ) ) ;
#6278=DIRECTION ( 'NONE',  ( 0.000000000000000000, 0.000000000000000000, -1.000000000000000000 ) ) ;
#6286=LINE ( 'NONE', #2118, #8780 ) ;
#6287=EDGE_CURVE ( 'NONE', #3376, #2611, #2861, .T. ) ;
#6294=EDGE_CURVE ( 'NONE', #69, #3614, #9037, .T. ) ;
#6297=LINE ( 'NONE', #2948, #8649 ) ;
#6299=CARTESIAN_POINT ( 'NONE',  ( 0.000000000000000000, -8.528980942125402365, 0.000000000000000000 ) ) ;
#6309=CARTESIAN_POINT ( 'NONE',  ( 17.40975659021752975, 3.343749999044085097, -17.40975659021752975 ) ) ;
#6316=CARTESIAN_POINT ( 'NONE',  ( -24.62111388750000174, 1.656249999044084431, -10.19839929293506131 ) ) ;
#6343=CARTESIAN_POINT ( 'NONE',  ( -10.35533905932737575, 3.312500000000000000, -25.00000000000000000 ) ) ;
#6357=DIRECTION ( 'NONE',  ( -0.000000000000000000, 1.000000000000000000, -0.000000000000000000 ) ) ;
#6359=CARTESIAN_POINT ( 'NONE',  ( -21.06539724162749394, 5.000000000000003553, 12.88420918705474705 ) ) ;
#6365=DIRECTION ( 'NONE',  ( -0.000000000000000000, 1.000000000000000000, -0.000000000000000000 ) ) ;
#6367=CARTESIAN_POINT ( 'NONE',  ( -24.62111388750000884, 1.781249999044084875, 10.19839929293505421 ) ) ;
#6368=CARTESIAN_POINT ( 'NONE',  ( 10.35533905932737930, 0.1874999999999999722, -25.00000000000000000 ) ) ;
#6376=CARTESIAN_POINT ( 'NONE',  ( 10.19839929293505953, 1.406249999044084653, -24.62111388750000174 ) ) ;
#6389=CARTESIAN_POINT ( 'NONE',  ( -4.592425496802574367E-15, 0.7500000000000000000, 25.00000000000000000 ) ) ;
#6398=ORIENTED_EDGE ( 'NONE', *, *, #10577, .T. ) ;
#6405=DIRECTION ( 'NONE',  ( 0.000000000000000000, -1.000000000000000000, 0.000000000000000000 ) ) ;
#6419=LINE ( 'NONE', #6466, #7287 ) ;
#6421=CARTESIAN_POINT ( 'NONE',  ( -17.40975659021753330, 2.843749999044085097, 17.40975659021752975 ) ) ;
#6426=ORIENTED_EDGE ( 'NONE', *, *, #50, .T. ) ;
#6429=CARTESIAN_POINT ( 'NONE',  ( -25.00000000000001421, 4.174999998088169129, 10.35533905932737397 ) ) ;
#6430=CARTESIAN_POINT ( 'NONE',  ( 10.19839929293505953, 4.406249999044084653, -24.62111388750000174 ) ) ;
#6463=VERTEX_POINT ( 'NONE', #9202 ) ;
#6466=CARTESIAN_POINT ( 'NONE',  ( 3.050810944027392283E-15, -58.00000000000000000, -24.91176187412963117 ) ) ;
#6474=CARTESIAN_POINT ( 'NONE',  ( -17.67766952966368876, 2.987499998088169129, -17.67766952966369232 ) ) ;
#6484=COLOUR_RGB ( '', 0.09019608, 0.27058824, 0.51372549) ;
#6493=CARTESIAN_POINT ( 'NONE',  ( -17.40975659021752975, 2.593749999044084653, -17.40975659021752975 ) ) ;
#6494=CYLINDRICAL_SURFACE ( 'NONE', #1634, 25.00000000000000000 ) ;
#6497=ORIENTED_EDGE ( 'NONE', *, *, #5661, .T. ) ;
#6504=DIRECTION ( 'NONE',  ( 0.8660254037844402619, -0.4999999999999970579, 0.000000000000000000 ) ) ;
#6509=FILL_AREA_STYLE_COLOUR ( '', #4785 ) ;
#6520=EDGE_CURVE ( 'NONE', #9493, #5323, #8933, .T. ) ;
#6524=CARTESIAN_POINT ( 'NONE',  ( -17.67766952966368876, 3.987499998088168685, -17.67766952966369232 ) ) ;
#6538=VERTEX_POINT ( 'NONE', #8925 ) ;
#6547=CARTESIAN_POINT ( 'NONE',  ( -24.62111388750000174, 1.718749999044084431, -3.015216831376932151E-15 ) ) ;
#6548=DIRECTION ( 'NONE',  ( 4.188538737677001009E-17, -0.9396926207859082059, 0.3420201433256694901 ) ) ;
#6550=VECTOR ( 'NONE', #2958, 1000.000000000000000 ) ;
#6552=AXIS2_PLACEMENT_3D ( 'NONE', #10305, #3668, #4525 ) ;
#6564=FILL_AREA_STYLE ('',( #6509 ) ) ;
#6570=FACE_BOUND ( 'NONE', #1222, .T. ) ;
#6575=VERTEX_POINT ( 'NONE', #8156 ) ;
#6580=CARTESIAN_POINT ( 'NONE',  ( 10.35533905932738286, 4.424999998088169129, 24.99999999999999645 ) ) ;
#6586=( NAMED_UNIT ( * ) SI_UNIT ( $, .STERADIAN. ) SOLID_ANGLE_UNIT ( ) );
#6596=VERTEX_POINT ( 'NONE', #1361 ) ;
#6597=EDGE_LOOP ( 'NONE', ( #4914, #5277, #8207, #10311 ) ) ;
#6605=CARTESIAN_POINT ( 'NONE',  ( 24.62111388749999463, 4.156249999044083765, 10.19839929293507730 ) ) ;
#6606=FACE_OUTER_BOUND ( 'NONE', #6198, .T. ) ;
#6608=ORIENTED_EDGE ( 'NONE', *, *, #4644, .F. ) ;
#6614=DIRECTION ( 'NONE',  ( 0.000000000000000000, -1.000000000000000000, 0.000000000000000000 ) ) ;
#6621=CARTESIAN_POINT ( 'NONE',  ( -24.62111388750000884, 0.9562499990440846975, 10.19839929293505421 ) ) ;
#6631=CARTESIAN_POINT ( 'NONE',  ( 10.19839929293505953, 0.5812499990440844755, -24.62111388750000174 ) ) ;
#6637=( LENGTH_UNIT ( ) NAMED_UNIT ( * ) SI_UNIT ( .MILLI., .METRE. ) );
#6643=ORIENTED_EDGE ( 'NONE', *, *, #2543, .F. ) ;
#6655=CARTESIAN_POINT ( 'NONE',  ( 25.00000000000000000, 4.612499998088169129, 0.000000000000000000 ) ) ;
#6657=CARTESIAN_POINT ( 'NONE',  ( 1.507608415688466075E-15, 0.4687499990440845421, -24.62111388750000174 ) ) ;
#6658=DIRECTION ( 'NONE',  ( 0.000000000000000000, 0.000000000000000000, -1.000000000000000000 ) ) ;
#6668=ADVANCED_FACE ( 'NONE', ( #1262 ), #7999, .T. ) ;
#6671=CARTESIAN_POINT ( 'NONE',  ( 5.592313892344211723, 5.000000000000000000, 23.99629895547188951 ) ) ;
#6684=CARTESIAN_POINT ( 'NONE',  ( 1.530808498934191521E-15, 4.250000000000000000, -25.00000000000000000 ) ) ;
#6687=CARTESIAN_POINT ( 'NONE',  ( 1.530808498934191521E-15, 3.250000000000000444, -25.00000000000000000 ) ) ;
#6692=CARTESIAN_POINT ( 'NONE',  ( 17.40975659021752620, 3.268749999044084475, 17.40975659021753330 ) ) ;
#6713=CARTESIAN_POINT ( 'NONE',  ( -16.34320696848747190, 5.000000000000000888, 18.55420638975051517 ) ) ;
#6715=CARTESIAN_POINT ( 'NONE',  ( 10.19839929293506486, 1.031249999044084653, 24.62111388749999819 ) ) ;
#6730=CARTESIAN_POINT ( 'NONE',  ( 16.80656569248275289, 5.000000000000001776, 18.21376690724898850 ) ) ;
#6746=CARTESIAN_POINT ( 'NONE',  ( -24.62111388750000174, 2.893749999044084475, -3.015216831376932151E-15 ) ) ;
#6767=CARTESIAN_POINT ( 'NONE',  ( -24.62111388750000174, 0.6562499990440846531, -10.19839929293506131 ) ) ;
#6776=AXIS2_PLACEMENT_3D ( 'NONE', #8214, #9057, #7385 ) ;
#6777=CARTESIAN_POINT ( 'NONE',  ( 25.00000000000000000, -2.710505431213761085E-17, 0.000000000000000000 ) ) ;
#6786=CARTESIAN_POINT ( 'NONE',  ( 2.694222958124177204E-15, -0.5289809421253948152, 22.00000000000000355 ) ) ;
#6795=ORIENTED_EDGE ( 'NONE', *, *, #2925, .T. ) ;
#6796=FACE_OUTER_BOUND ( 'NONE', #7367, .T. ) ;
#6798=LINE ( 'NONE', #10155, #2002 ) ;
#6803=CARTESIAN_POINT ( 'NONE',  ( -10.19839929293505776, 2.706249999044084475, -24.62111388750000174 ) ) ;
#6810=CARTESIAN_POINT ( 'NONE',  ( 10.35533905932738286, 1.424999998088169129, 24.99999999999999645 ) ) ;
#6819=CARTESIAN_POINT ( 'NONE',  ( -24.62111388750000174, 3.831249999044084920, -10.19839929293506131 ) ) ;
#6827=CARTESIAN_POINT ( 'NONE',  ( -10.35533905932739174, 2.687500000000000444, 24.99999999999999289 ) ) ;
#6828=CARTESIAN_POINT ( 'NONE',  ( -25.00000000000001066, 3.174999998088169573, 10.35533905932737397 ) ) ;
#6832=ORIENTED_EDGE ( 'NONE', *, *, #8009, .F. ) ;
#6843=CARTESIAN_POINT ( 'NONE',  ( -4.592425496802574367E-15, 4.750000000000000000, 25.00000000000000000 ) ) ;
#6846=CARTESIAN_POINT ( 'NONE',  ( 0.000000000000000000, -55.00000000000000000, 0.000000000000000000 ) ) ;
#6852=B_SPLINE_CURVE_WITH_KNOTS ( 'NONE', 3,
 ( #4168, #5995, #1507, #2486, #3310, #1561, #10071, #6713, #4888, #5883 ),
 .UNSPECIFIED., .F., .F.,
 ( 4, 2, 2, 2, 4 ),
 ( 0.000000000000000000, 0.006815791626871553661, 0.01363158325374310732, 0.02044737488061466185, 0.02726316650748621465 ),
 .UNSPECIFIED. ) ;
#6856=CARTESIAN_POINT ( 'NONE',  ( 17.40975659021752975, 0.5187499990440846975, -17.40975659021752975 ) ) ;
#6857=CARTESIAN_POINT ( 'NONE',  ( 10.19839929293506486, 3.206249999044084031, 24.62111388749999819 ) ) ;
#6865=CARTESIAN_POINT ( 'NONE',  ( 25.00000000000000000, 0.6749999980881690176, -10.35533905932737753 ) ) ;
#6867=CARTESIAN_POINT ( 'NONE',  ( -25.00000000000000000, 4.437500000000000888, -10.35533905932738108 ) ) ;
#6876=CARTESIAN_POINT ( 'NONE',  ( -24.62111388750000884, 0.7812499990440845421, 10.19839929293505421 ) ) ;
#6884=CARTESIAN_POINT ( 'NONE',  ( 17.67766952966368521, 4.875000000000000000, 17.67766952966369232 ) ) ;
#6896=AXIS2_PLACEMENT_3D ( 'NONE', #850, #4061, #8463 ) ;
#6911=CARTESIAN_POINT ( 'NONE',  ( -10.35533905932741128, 4.924999998088170905, -24.99999999999996803 ) ) ;
#6914=CARTESIAN_POINT ( 'NONE',  ( -24.62111388750000174, 4.893749999044084475, -3.015216831376932151E-15 ) ) ;
#6915=EDGE_LOOP ( 'NONE', ( #4153, #1359, #10624 ) ) ;
#6921=CARTESIAN_POINT ( 'NONE',  ( -17.40975659021753330, 3.018749999044084475, 17.40975659021752975 ) ) ;
#6927=CARTESIAN_POINT ( 'NONE',  ( 3.234507963899495005E-15, -58.00000000000000000, 24.91176187412963117 ) ) ;
#6932=CARTESIAN_POINT ( 'NONE',  ( 25.00000000000000000, 3.062500000000000000, -10.35533905932737753 ) ) ;
#6937=CARTESIAN_POINT ( 'NONE',  ( 24.62111388750000174, 4.456249999044085364, -10.19839929293505776 ) ) ;
#6943=ADVANCED_FACE ( 'NONE', ( #262 ), #5407, .F. ) ;
#6944=PLANE ( 'NONE',  #6552 ) ;
#6947=CARTESIAN_POINT ( 'NONE',  ( -25.00000000000000000, 1.500000000000000000, -3.061616997868383043E-15 ) ) ;
#6973=CARTESIAN_POINT ( 'NONE',  ( 17.40975659021752975, 2.518749999044084475, -17.40975659021752975 ) ) ;
#6974=CARTESIAN_POINT ( 'NONE',  ( 0.000000000000000000, -8.000000000000000000, -27.91176187412962761 ) ) ;
#6986=CARTESIAN_POINT ( 'NONE',  ( 17.67766952966369232, 0.7374999980881691286, -17.67766952966369232 ) ) ;
#6987=CARTESIAN_POINT ( 'NONE',  ( -17.67766952966368876, 3.375000000000000000, -17.67766952966369232 ) ) ;
#6992=CARTESIAN_POINT ( 'NONE',  ( 10.19839929293506486, 3.206249999044084031, 24.62111388749999819 ) ) ;
#7007=EDGE_CURVE ( 'NONE', #2886, #2611, #2224, .T. ) ;
#7010=DIRECTION ( 'NONE',  ( -0.000000000000000000, 1.000000000000000000, -0.000000000000000000 ) ) ;
#7015=ORIENTED_EDGE ( 'NONE', *, *, #10438, .F. ) ;
#7021=CARTESIAN_POINT ( 'NONE',  ( 24.62111388749999108, 2.331249999044084475, 10.19839929293507730 ) ) ;
#7028=ADVANCED_FACE ( 'NONE', ( #7986 ), #48, .T. ) ;
#7030=VECTOR ( 'NONE', #5917, 1000.000000000000000 ) ;
#7036=VECTOR ( 'NONE', #3442, 1000.000000000000000 ) ;
#7037=CARTESIAN_POINT ( 'NONE',  ( -10.19839929293507375, 0.9062499990440844311, 24.62111388749999108 ) ) ;
#7040=AXIS2_PLACEMENT_3D ( 'NONE', #1904, #3431, #7048 ) ;
#7044=CARTESIAN_POINT ( 'NONE',  ( 17.40975659021752620, 4.093749999044084653, 17.40975659021753330 ) ) ;
#7048=DIRECTION ( 'NONE',  ( 1.000000000000000000, 0.000000000000000000, 0.000000000000000000 ) ) ;
#7053=CARTESIAN_POINT ( 'NONE',  ( -25.00000000000000000, 2.437500000000000444, -10.35533905932738108 ) ) ;
#7061=PRODUCT_DEFINITION_FORMATION_WITH_SPECIFIED_SOURCE ( 'ANY', '', #4420, .NOT_KNOWN. ) ;
#7063=CARTESIAN_POINT ( 'NONE',  ( 0.000000000000000000, -58.00000000000000000, 0.000000000000000000 ) ) ;
#7068=ORIENTED_EDGE ( 'NONE', *, *, #9694, .T. ) ;
#7074=CARTESIAN_POINT ( 'NONE',  ( 10.19839929293505953, 3.581249999044085364, -24.62111388750000174 ) ) ;
#7092=CARTESIAN_POINT ( 'NONE',  ( 24.62111388749999108, 1.156249999044084431, 10.19839929293507730 ) ) ;
#7093=DIRECTION ( 'NONE',  ( 0.000000000000000000, -1.000000000000000000, 0.000000000000000000 ) ) ;
#7099=CARTESIAN_POINT ( 'NONE',  ( 24.62111388750000174, 2.281249999044085541, -10.19839929293505776 ) ) ;
#7111=DIRECTION ( 'NONE',  ( -1.224646799147353454E-16, 0.000000000000000000, -1.000000000000000000 ) ) ;
#7117=DIRECTION ( 'NONE',  ( 0.000000000000000000, -1.000000000000000000, 0.000000000000000000 ) ) ;
#7124=CARTESIAN_POINT ( 'NONE',  ( -24.62111388750000174, 2.893749999044084475, -3.015216831376932151E-15 ) ) ;
#7136=CARTESIAN_POINT ( 'NONE',  ( 24.62111388749999463, 5.331249999044085364, 10.19839929293507730 ) ) ;
#7144=CARTESIAN_POINT ( 'NONE',  ( -24.62111388750000884, 3.781249999044084653, 10.19839929293505421 ) ) ;
#7150=CARTESIAN_POINT ( 'NONE',  ( -24.62111388750000174, 3.656249999044084653, -10.19839929293506131 ) ) ;
#7157=CARTESIAN_POINT ( 'NONE',  ( -10.35533905932737575, 2.312500000000000888, -25.00000000000000000 ) ) ;
#7158=ORIENTED_EDGE ( 'NONE', *, *, #8125, .F. ) ;
#7168=CARTESIAN_POINT ( 'NONE',  ( -4.592425496802574367E-15, 3.750000000000000000, 25.00000000000000000 ) ) ;
#7169=ORIENTED_EDGE ( 'NONE', *, *, #9789, .T. ) ;
#7171=ORIENTED_EDGE ( 'NONE', *, *, #4857, .T. ) ;
#7173=DIRECTION ( 'NONE',  ( 0.000000000000000000, 0.000000000000000000, -1.000000000000000000 ) ) ;
#7175=DIRECTION ( 'NONE',  ( -0.000000000000000000, 1.000000000000000000, -0.000000000000000000 ) ) ;
#7179=EDGE_LOOP ( 'NONE', ( #2709, #2210, #4687, #8586 ) ) ;
#7180=DIRECTION ( 'NONE',  ( -1.000000000000000000, -0.000000000000000000, -0.000000000000000000 ) ) ;
#7181=DIRECTION ( 'NONE',  ( 0.000000000000000000, 0.000000000000000000, -1.000000000000000000 ) ) ;
#7187=CARTESIAN_POINT ( 'NONE',  ( 24.62111388750000174, 4.218749999044084653, 0.000000000000000000 ) ) ;
#7191=CIRCLE ( 'NONE', #9666, 25.00000000000000000 ) ;
#7192=CARTESIAN_POINT ( 'NONE',  ( -10.19839929293507552, 2.906249999044085541, 24.62111388749999463 ) ) ;
#7211=LINE ( 'NONE', #7359, #7630 ) ;
#7232=CARTESIAN_POINT ( 'NONE',  ( -24.62111388750000174, 1.718749999044084431, -3.015216831376932151E-15 ) ) ;
#7242=CARTESIAN_POINT ( 'NONE',  ( -24.62111388750000884, 4.781249999044083765, 10.19839929293505421 ) ) ;
#7250=EDGE_LOOP ( 'NONE', ( #1688, #3177, #4002, #914 ) ) ;
#7258=EDGE_CURVE ( 'NONE', #9966, #10861, #7450, .T. ) ;
#7273=VECTOR ( 'NONE', #3406, 1000.000000000000000 ) ;
#7287=VECTOR ( 'NONE', #6365, 1000.000000000000000 ) ;
#7288=CARTESIAN_POINT ( 'NONE',  ( 17.40975659021752620, 4.093749999044084653, 17.40975659021753330 ) ) ;
#7294=CARTESIAN_POINT ( 'NONE',  ( -25.00000000000000000, 3.112499998088169129, -3.061616997868383043E-15 ) ) ;
#7305=CARTESIAN_POINT ( 'NONE',  ( 17.67766952966368521, 3.875000000000000000, 17.67766952966369232 ) ) ;
#7307=CARTESIAN_POINT ( 'NONE',  ( 17.67766952966368521, 1.487499998088169129, 17.67766952966369232 ) ) ;
#7308=CARTESIAN_POINT ( 'NONE',  ( 0.000000000000000000, 5.000000000000000000, 0.000000000000000000 ) ) ;
#7311=CARTESIAN_POINT ( 'NONE',  ( -24.62111388750000884, 1.781249999044084431, 10.19839929293505421 ) ) ;
#7317=DIRECTION ( 'NONE',  ( 0.000000000000000000, 0.000000000000000000, -1.000000000000000000 ) ) ;
#7321=ADVANCED_FACE ( 'NONE', ( #3765 ), #1891, .T. ) ;
#7331=CARTESIAN_POINT ( 'NONE',  ( 17.67766952966369232, 3.737499998088169573, -17.67766952966369232 ) ) ;
#7341=ADVANCED_FACE ( 'NONE', ( #6570, #2365 ), #708, .F. ) ;
#7342=CARTESIAN_POINT ( 'NONE',  ( -10.35533905932739174, 5.299999998088169129, 24.99999999999999289 ) ) ;
#7348=DIRECTION ( 'NONE',  ( 0.000000000000000000, -1.000000000000000000, 0.000000000000000000 ) ) ;
#7358=ORIENTED_EDGE ( 'NONE', *, *, #3248, .F. ) ;
#7359=CARTESIAN_POINT ( 'NONE',  ( 3.061616997868383043E-15, 5.000000000000000000, 25.00000000000000000 ) ) ;
#7362=CARTESIAN_POINT ( 'NONE',  ( -10.19839929293505776, 3.531249999044084653, -24.62111388750000174 ) ) ;
#7363=CARTESIAN_POINT ( 'NONE',  ( -25.00000000000000000, 3.500000000000000000, -3.061616997868383043E-15 ) ) ;
#7367=EDGE_LOOP ( 'NONE', ( #7983, #2953 ) ) ;
#7371=DIRECTION ( 'NONE',  ( 0.000000000000000000, 0.000000000000000000, -1.000000000000000000 ) ) ;
#7385=DIRECTION ( 'NONE',  ( 0.000000000000000000, -0.000000000000000000, -1.000000000000000000 ) ) ;
#7389=EDGE_CURVE ( 'NONE', #8219, #10861, #6419, .T. ) ;
#7393=CONICAL_SURFACE ( 'NONE', #3731, 22.18092213764227694, 0.3490658503988666728 ) ;
#7396=CARTESIAN_POINT ( 'NONE',  ( 24.62111388749999463, 1.331249999044084475, 10.19839929293507730 ) ) ;
#7403=DIRECTION ( 'NONE',  ( 0.000000000000000000, -1.000000000000000000, 0.000000000000000000 ) ) ;
#7417=ORIENTED_EDGE ( 'NONE', *, *, #319, .F. ) ;
#7421=CARTESIAN_POINT ( 'NONE',  ( 17.40975659021752975, 3.343749999044085097, -17.40975659021752975 ) ) ;
#7425=VECTOR ( 'NONE', #3151, 1000.000000000000114 ) ;
#7428=DIRECTION ( 'NONE',  ( 0.000000000000000000, -1.000000000000000000, 0.000000000000000000 ) ) ;
#7432=LINE ( 'NONE', #9044, #1817 ) ;
#7449=( BOUNDED_CURVE ( )  B_SPLINE_CURVE ( 2, ( #2738, #9495, #4489, #273, #3635, #5004, #9076, #10734, #10 ),
 .UNSPECIFIED., .F., .F. ) 
 B_SPLINE_CURVE_WITH_KNOTS ( ( 3, 2, 2, 2, 3 ),
 ( 0.5500000000000000444, 0.5749999999999999556, 0.5999999999999999778, 0.6250000000000000000, 0.6500000000000000222 ),
 .UNSPECIFIED. ) 
 CURVE ( )  GEOMETRIC_REPRESENTATION_ITEM ( )  RATIONAL_B_SPLINE_CURVE ( ( 1.000000000000000000, 0.9238795325112867385, 1.000000000000000000, 0.9238795325112867385, 1.000000000000000000, 0.9238795325112867385, 1.000000000000000000, 0.9238795325112867385, 1.000000000000000000 ) ) 
 REPRESENTATION_ITEM ( '' )  );
#7450=CIRCLE ( 'NONE', #2687, 24.91176187412963117 ) ;
#7454=CARTESIAN_POINT ( 'NONE',  ( -4.592425496802574367E-15, 5.362499998088169129, 25.00000000000000000 ) ) ;
#7459=ORIENTED_EDGE ( 'NONE', *, *, #2543, .T. ) ;
#7467=EDGE_CURVE ( 'NONE', #9967, #57, #4522, .T. ) ;
#7469=AXIS2_PLACEMENT_3D ( 'NONE', #9257, #1702, #10154 ) ;
#7479=CARTESIAN_POINT ( 'NONE',  ( 17.40975659021752620, 1.093749999044084653, 17.40975659021753330 ) ) ;
#7480=DIRECTION ( 'NONE',  ( 0.000000000000000000, -1.000000000000000000, 0.000000000000000000 ) ) ;
#7481=CARTESIAN_POINT ( 'NONE',  ( -10.19839929293507552, 2.906249999044085541, 24.62111388749999463 ) ) ;
#7487=VERTEX_POINT ( 'NONE', #6684 ) ;
#7490=CARTESIAN_POINT ( 'NONE',  ( 0.000000000000000000, 5.000000000000000000, -25.00000000000000000 ) ) ;
#7493=CARTESIAN_POINT ( 'NONE',  ( 8.318560929346013211, 5.000000000000000000, 23.22693844957334619 ) ) ;
#7495=ORIENTED_EDGE ( 'NONE', *, *, #8684, .F. ) ;
#7497=DIRECTION ( 'NONE',  ( 0.000000000000000000, 0.000000000000000000, -1.000000000000000000 ) ) ;
#7509=CARTESIAN_POINT ( 'NONE',  ( 17.40975659021752620, 4.268749999044084475, 17.40975659021753330 ) ) ;
#7510=CARTESIAN_POINT ( 'NONE',  ( 0.000000000000000000, 5.000000000000000000, -25.00000000000000000 ) ) ;
#7520=( BOUNDED_CURVE ( )  B_SPLINE_CURVE ( 2, ( #4815, #8175, #5692, #9207, #9873, #1535, #657, #1652, #10766 ),
 .UNSPECIFIED., .F., .F. ) 
 B_SPLINE_CURVE_WITH_KNOTS ( ( 3, 2, 2, 2, 3 ),
 ( 0.2500000000000000000, 0.2750000000000000222, 0.3000000000000000444, 0.3250000000000000666, 0.3500000000000000333 ),
 .UNSPECIFIED. ) 
 CURVE ( )  GEOMETRIC_REPRESENTATION_ITEM ( )  RATIONAL_B_SPLINE_CURVE ( ( 1.000000000000000000, 0.9238795325112867385, 1.000000000000000000, 0.9238795325112867385, 1.000000000000000000, 0.9238795325112867385, 1.000000000000000000, 0.9238795325112865164, 1.000000000000000222 ) ) 
 REPRESENTATION_ITEM ( '' )  );
#7525=ADVANCED_FACE ( 'NONE', ( #2411 ), #9984, .T. ) ;
#7531=CARTESIAN_POINT ( 'NONE',  ( 17.40975659021752620, 2.093749999044084653, 17.40975659021753330 ) ) ;
#7545=CARTESIAN_POINT ( 'NONE',  ( 24.33865891316265362, 5.000000000000000000, 5.618519342023028607 ) ) ;
#7550=ORIENTED_EDGE ( 'NONE', *, *, #1322, .T. ) ;
#7576=CARTESIAN_POINT ( 'NONE',  ( 24.62111388750000174, 2.393749999044084475, 0.000000000000000000 ) ) ;
#7582=EDGE_LOOP ( 'NONE', ( #4485, #9213, #10875, #7495 ) ) ;
#7584=CARTESIAN_POINT ( 'NONE',  ( 24.62111388750000174, 0.3062499990440845643, 0.000000000000000000 ) ) ;
#7598=CARTESIAN_POINT ( 'NONE',  ( 0.000000000000000000, 5.000000000000000000, 0.000000000000000000 ) ) ;
#7605=VECTOR ( 'NONE', #8362, 1000.000000000000000 ) ;
#7610=LINE ( 'NONE', #10333, #7273 ) ;
#7617=FACE_OUTER_BOUND ( 'NONE', #4854, .T. ) ;
#7619=CARTESIAN_POINT ( 'NONE',  ( 0.000000000000000000, -58.00000000000000000, 24.91176187412963117 ) ) ;
#7625=VECTOR ( 'NONE', #6548, 999.9999999999998863 ) ;
#7630=VECTOR ( 'NONE', #9904, 1000.000000000000000 ) ;
#7636=CARTESIAN_POINT ( 'NONE',  ( 17.40975659021752975, 4.518749999044085364, -17.40975659021752975 ) ) ;
#7646=CARTESIAN_POINT ( 'NONE',  ( -24.62111388750000174, 4.718749999044084653, -3.015216831376932151E-15 ) ) ;
#7647=CARTESIAN_POINT ( 'NONE',  ( -17.67766952966368876, 2.987499998088169129, -17.67766952966369232 ) ) ;
#7657=CARTESIAN_POINT ( 'NONE',  ( 1.530808498934191521E-15, 2.250000000000000444, -25.00000000000000000 ) ) ;
#7660=LINE ( 'NONE', #7936, #1083 ) ;
#7661=CARTESIAN_POINT ( 'NONE',  ( 23.96357173135144691, 5.000000000000001776, 6.992167731761885996 ) ) ;
#7677=CARTESIAN_POINT ( 'NONE',  ( -24.62111388750000884, 2.956249999044084475, 10.19839929293505421 ) ) ;
#7682=EDGE_CURVE ( 'NONE', #6575, #39, #9502, .T. ) ;
#7687=CARTESIAN_POINT ( 'NONE',  ( -17.67766952966368876, 1.987499998088169129, -17.67766952966369232 ) ) ;
#7689=CARTESIAN_POINT ( 'NONE',  ( 1.530808498934191521E-15, 4.250000000000000000, -25.00000000000000000 ) ) ;
#7696=CARTESIAN_POINT ( 'NONE',  ( -24.62111388750000884, 4.956249999044084475, 10.19839929293505421 ) ) ;
#7724=CARTESIAN_POINT ( 'NONE',  ( 1.530808498934191521E-15, 4.250000000000000000, -25.00000000000000000 ) ) ;
#7725=CARTESIAN_POINT ( 'NONE',  ( 1.507608415688466075E-15, 4.643749999044084475, -24.62111388750000174 ) ) ;
#7735=CARTESIAN_POINT ( 'NONE',  ( -24.62111388750000884, 0.9562499990440846975, 10.19839929293505421 ) ) ;
#7745=CARTESIAN_POINT ( 'NONE',  ( 25.00000000000000000, 2.674999998088169129, -10.35533905932737753 ) ) ;
#7747=CARTESIAN_POINT ( 'NONE',  ( -10.35533905932737575, 3.312500000000000000, -25.00000000000000000 ) ) ;
#7750=ORIENTED_EDGE ( 'NONE', *, *, #4788, .F. ) ;
#7752=CARTESIAN_POINT ( 'NONE',  ( -17.40975659021752975, 2.768749999044084475, -17.40975659021752975 ) ) ;
#7762=CARTESIAN_POINT ( 'NONE',  ( 24.99999999999999289, 4.937500000000001776, 10.35533905932739529 ) ) ;
#7763=CARTESIAN_POINT ( 'NONE',  ( 24.62111388750000174, 5.218749999044084653, 0.000000000000000000 ) ) ;
#7764=CARTESIAN_POINT ( 'NONE',  ( -4.592425496802574367E-15, 2.750000000000000000, 25.00000000000000000 ) ) ;
#7769=PRODUCT_DEFINITION_SHAPE ( 'NONE', 'NONE',  #10146 ) ;
#7777=DIRECTION ( 'NONE',  ( 0.000000000000000000, -1.000000000000000000, 0.000000000000000000 ) ) ;
#7788=CARTESIAN_POINT ( 'NONE',  ( -17.40975659021752975, 4.768749999044084475, -17.40975659021752975 ) ) ;
#7796=CARTESIAN_POINT ( 'NONE',  ( -17.40975659021752975, 1.768749999044084475, -17.40975659021752975 ) ) ;
#7803=CARTESIAN_POINT ( 'NONE',  ( 17.40975659021752975, 0.3437499990440845421, -17.40975659021752975 ) ) ;
#7812=CARTESIAN_POINT ( 'NONE',  ( -4.522825247065398226E-15, 5.143749999044084475, 24.62111388750000174 ) ) ;
#7823=CARTESIAN_POINT ( 'NONE',  ( 1.530808498934191521E-15, 4.862499998088169129, -25.00000000000000000 ) ) ;
#7824=CARTESIAN_POINT ( 'NONE',  ( -25.00000000000000000, 0.5000000000000000000, -3.061616997868383043E-15 ) ) ;
#7838=DIRECTION ( 'NONE',  ( 0.000000000000000000, 0.000000000000000000, -1.000000000000000000 ) ) ;
#7851=CARTESIAN_POINT ( 'NONE',  ( 10.19839929293505953, 1.581249999044084475, -24.62111388750000174 ) ) ;
#7859=CARTESIAN_POINT ( 'NONE',  ( -24.78791250444086458, 5.000000000000001776, -1.973611014893982940 ) ) ;
#7866=CARTESIAN_POINT ( 'NONE',  ( 17.67766952966368521, 1.487499998088169129, 17.67766952966369232 ) ) ;
#7869=CARTESIAN_POINT ( 'NONE',  ( -24.62111388750000174, 1.893749999044084475, -3.015216831376932151E-15 ) ) ;
#7873=CARTESIAN_POINT ( 'NONE',  ( 17.40975659021752975, 1.343749999044084653, -17.40975659021752975 ) ) ;
#7880=CARTESIAN_POINT ( 'NONE',  ( -10.35533905932739174, 4.687500000000000888, 24.99999999999999289 ) ) ;
#7883=ORIENTED_EDGE ( 'NONE', *, *, #4579, .F. ) ;
#7896=( BOUNDED_CURVE ( )  B_SPLINE_CURVE ( 2, ( #630, #6343, #9029, #2186, #7363, #1463, #3153, #10638, #7168 ),
 .UNSPECIFIED., .F., .F. ) 
 B_SPLINE_CURVE_WITH_KNOTS ( ( 3, 2, 2, 2, 3 ),
 ( 0.6500000000000000222, 0.6750000000000000444, 0.6999999999999999556, 0.7249999999999999778, 0.7500000000000000000 ),
 .UNSPECIFIED. ) 
 CURVE ( )  GEOMETRIC_REPRESENTATION_ITEM ( )  RATIONAL_B_SPLINE_CURVE ( ( 1.000000000000000000, 0.9238795325112867385, 1.000000000000000000, 0.9238795325112867385, 1.000000000000000000, 0.9238795325112867385, 1.000000000000000000, 0.9238795325112867385, 1.000000000000000000 ) ) 
 REPRESENTATION_ITEM ( '' )  );
#7902=CARTESIAN_POINT ( 'NONE',  ( 17.40975659021752620, 1.268749999044084475, 17.40975659021753330 ) ) ;
#7916=CARTESIAN_POINT ( 'NONE',  ( -17.40975659021753330, 4.843749999044083765, 17.40975659021752975 ) ) ;
#7921=CARTESIAN_POINT ( 'NONE',  ( 10.19839929293506486, 2.031249999044084653, 24.62111388749999819 ) ) ;
#7926=DIRECTION ( 'NONE',  ( 0.000000000000000000, -1.000000000000000000, 0.000000000000000000 ) ) ;
#7927=CARTESIAN_POINT ( 'NONE',  ( -17.67766952966368876, 2.375000000000000000, -17.67766952966369232 ) ) ;
#7928=CARTESIAN_POINT ( 'NONE',  ( -17.67766952966369232, 4.625000000000000000, 17.67766952966368876 ) ) ;
#7935=EDGE_CURVE ( 'NONE', #1367, #8849, #2518, .T. ) ;
#7936=CARTESIAN_POINT ( 'NONE',  ( 3.061616997868383043E-15, 5.000000000000000000, 25.00000000000000000 ) ) ;
#7943=ORIENTED_EDGE ( 'NONE', *, *, #5661, .F. ) ;
#7945=CARTESIAN_POINT ( 'NONE',  ( 10.19839929293506486, 4.206249999044083587, 24.62111388749999819 ) ) ;
#7959=CARTESIAN_POINT ( 'NONE',  ( -24.62111388750000174, 4.831249999044084475, -10.19839929293506131 ) ) ;
#7961=CARTESIAN_POINT ( 'NONE',  ( -24.64992079640905587, 4.999999999999998224, -3.388298626009401460 ) ) ;
#7964=LINE ( 'NONE', #341, #6550 ) ;
#7966=ORIENTED_EDGE ( 'NONE', *, *, #7258, .F. ) ;
#7967=CARTESIAN_POINT ( 'NONE',  ( 24.62111388750000174, 2.281249999044085541, -10.19839929293505776 ) ) ;
#7973=CARTESIAN_POINT ( 'NONE',  ( 24.62111388750000174, 4.218749999044084653, 0.000000000000000000 ) ) ;
#7977=LINE ( 'NONE', #6277, #364 ) ;
#7980=CARTESIAN_POINT ( 'NONE',  ( 25.00000000000000000, 2.062500000000000000, -10.35533905932737753 ) ) ;
#7983=ORIENTED_EDGE ( 'NONE', *, *, #2523, .F. ) ;
#7985=DIRECTION ( 'NONE',  ( 1.000000000000000000, 0.000000000000000000, -1.224646799147353207E-16 ) ) ;
#7986=FACE_OUTER_BOUND ( 'NONE', #8560, .T. ) ;
#7997=EDGE_LOOP ( 'NONE', ( #1655, #8886, #1469, #1007 ) ) ;
#7999=CYLINDRICAL_SURFACE ( 'NONE', #2495, 25.00000000000000000 ) ;
#8000=CIRCLE ( 'NONE', #3208, 25.00000000000000000 ) ;
#8002=AXIS2_PLACEMENT_3D ( 'NONE', #7598, #2555, #25 ) ;
#8009=EDGE_CURVE ( 'NONE', #3376, #5115, #1822, .T. ) ;
#8014=VERTEX_POINT ( 'NONE', #6786 ) ;
#8017=CARTESIAN_POINT ( 'NONE',  ( 2.472467130856905282, 4.983902298070619352, 24.62111388750000174 ) ) ;
#8024=CARTESIAN_POINT ( 'NONE',  ( 24.62111388750000174, 3.281249999044085097, -10.19839929293505776 ) ) ;
#8047=DIRECTION ( 'NONE',  ( 0.000000000000000000, -1.000000000000000000, 0.000000000000000000 ) ) ;
#8053=CARTESIAN_POINT ( 'NONE',  ( -22.18568234790235039, 4.999999999999997335, -11.47449125965302841 ) ) ;
#8059=( GEOMETRIC_REPRESENTATION_CONTEXT ( 3 ) GLOBAL_UNCERTAINTY_ASSIGNED_CONTEXT ( ( #8356 ) ) GLOBAL_UNIT_ASSIGNED_CONTEXT ( ( #6637, #9995, #6586 ) ) REPRESENTATION_CONTEXT ( 'NONE', 'WORKASPACE' ) );
#8060=CARTESIAN_POINT ( 'NONE',  ( 24.62111388750000174, 2.218749999044084653, 0.000000000000000000 ) ) ;
#8061=CARTESIAN_POINT ( 'NONE',  ( 1.530808498934191521E-15, 0.2500000000000000000, -25.00000000000000000 ) ) ;
#8067=EDGE_CURVE ( 'NONE', #3676, #6596, #5541, .T. ) ;
#8069=CARTESIAN_POINT ( 'NONE',  ( -24.62111388750000174, 4.656249999044085541, -10.19839929293506131 ) ) ;
#8081=ORIENTED_EDGE ( 'NONE', *, *, #845, .T. ) ;
#8088=DIRECTION ( 'NONE',  ( 0.000000000000000000, -1.000000000000000000, 0.000000000000000000 ) ) ;
#8106=CARTESIAN_POINT ( 'NONE',  ( -4.592425496802574367E-15, 4.750000000000000000, 25.00000000000000000 ) ) ;
#8115=CARTESIAN_POINT ( 'NONE',  ( -17.40975659021752975, 3.593749999044084653, -17.40975659021752975 ) ) ;
#8116=CARTESIAN_POINT ( 'NONE',  ( 25.00000000000000000, 4.062500000000000000, -10.35533905932737753 ) ) ;
#8119=CIRCLE ( 'NONE', #10060, 24.91176187412963117 ) ;
#8121=CARTESIAN_POINT ( 'NONE',  ( 24.99999999999999289, 4.549999998088169129, 10.35533905932739529 ) ) ;
#8125=EDGE_CURVE ( 'NONE', #8014, #10892, #3591, .T. ) ;
#8133=EDGE_CURVE ( 'NONE', #4397, #8924, #5019, .T. ) ;
#8147=CARTESIAN_POINT ( 'NONE',  ( 0.000000000000000000, -1.026060429977008193, 0.000000000000000000 ) ) ;
#8152=ORIENTED_EDGE ( 'NONE', *, *, #256, .T. ) ;
#8156=CARTESIAN_POINT ( 'NONE',  ( 1.530808498934191521E-15, 1.250000000000000000, -25.00000000000000000 ) ) ;
#8164=ORIENTED_EDGE ( 'NONE', *, *, #6287, .T. ) ;
#8168=DIRECTION ( 'NONE',  ( 0.000000000000000000, -1.000000000000000000, 0.000000000000000000 ) ) ;
#8175=CARTESIAN_POINT ( 'NONE',  ( -10.35533905932737575, 1.312500000000000222, -25.00000000000000000 ) ) ;
#8180=CARTESIAN_POINT ( 'NONE',  ( -17.67766952966369232, 3.237499998088169573, 17.67766952966368876 ) ) ;
#8195=FACE_OUTER_BOUND ( 'NONE', #2189, .T. ) ;
#8196=CARTESIAN_POINT ( 'NONE',  ( -17.40975659021752975, 1.593749999044084431, -17.40975659021752975 ) ) ;
#8207=ORIENTED_EDGE ( 'NONE', *, *, #8407, .F. ) ;
#8208=ADVANCED_FACE ( 'NONE', ( #2837 ), #10481, .T. ) ;
#8214=CARTESIAN_POINT ( 'NONE',  ( 0.000000000000000000, 5.000000000000000000, 0.000000000000000000 ) ) ;
#8219=VERTEX_POINT ( 'NONE', #6124 ) ;
#8220=( BOUNDED_SURFACE ( )  B_SPLINE_SURFACE ( 1, 2, ( 
 ( #3465, #5969, #6856, #886, #4316, #164, #2631, #4255, #4370, #7735, #10335, #51, #3410, #10160, #10277, #2695, #950, #6028, #9388, #6091, #8614, #1059, #7796, #228, #7869, #293, #3658, #6156, #9522, #10868, #8457, #904, #7576, #4390, #2761, #2646, #6046, #9405, #7752, #5167, #9468, #2594, #3544, #10176, #9341, #6992, #1727, #1846, #1786, #5932, #245, #4454, #5103, #6107, #5988, #6819, #1021, #1900, #4271, #5229, #5281, #8516, #8572, #184, #4213, #6937, #7636, #969, #10297, #8629, #2539, #2711, #4333, #7696, #1078, #125, #7812, #3604, #9282, #10348, #6160 ),
 ( #9525, #3486, #5058, #8402, #844, #7, #3367, #6767, #10127, #6876, #10234, #72, #3427, #5391, #3825, #4566, #2970, #3721, #7873, #6376, #8691, #9682, #9730, #6316, #10514, #1138, #5334, #6218, #349, #7921, #10402, #3778, #1961, #7099, #2820, #10461, #503, #8747, #404, #2876, #4717, #2057, #9630, #7192, #5543, #3874, #1291, #6273, #5433, #8024, #4517, #8796, #10560, #4674, #2919, #7150, #296, #2105, #1235, #2159, #4618, #3661, #7044, #5483, #7973, #1186, #9578, #6430, #455, #8903, #1338, #8069, #8847, #7242, #2019, #10613, #3029, #9108, #3182, #8276, #1495 ) ),
 .UNSPECIFIED., .F., .F., .F. ) 
 B_SPLINE_SURFACE_WITH_KNOTS ( ( 2, 2 ),
 ( 3, 2, 2, 2, 2, 2, 2, 2, 2, 2, 2, 2, 2, 2, 2, 2, 2, 2, 2, 2, 2, 2, 2, 2, 2, 2, 2, 2, 2, 2, 2, 2, 2, 2, 2, 2, 2, 2, 2, 2, 3 ),
 ( 0.000000000000000000, 1.000000000000000000 ),
 ( 0.000000000000000000, 0.02500000000000000139, 0.05000000000000000278, 0.07499999999999999722, 0.1000000000000000056, 0.1250000000000000000, 0.1499999999999999944, 0.1749999999999999889, 0.2000000000000000111, 0.2250000000000000056, 0.2500000000000000000, 0.2750000000000000222, 0.2999999999999999889, 0.3250000000000000111, 0.3499999999999999778, 0.3750000000000000000, 0.4000000000000000222, 0.4249999999999999889, 0.4500000000000000111, 0.4749999999999999778, 0.5000000000000000000, 0.5250000000000000222, 0.5500000000000000444, 0.5749999999999999556, 0.5999999999999999778, 0.6250000000000000000, 0.6500000000000000222, 0.6750000000000000444, 0.6999999999999999556, 0.7249999999999999778, 0.7500000000000000000, 0.7750000000000000222, 0.8000000000000000444, 0.8249999999999999556, 0.8499999999999999778, 0.8750000000000000000, 0.9000000000000000222, 0.9250000000000000444, 0.9499999999999999556, 0.9749999999999999778, 1.000000000000000000 ),
 .UNSPECIFIED. ) 
 GEOMETRIC_REPRESENTATION_ITEM ( )  RATIONAL_B_SPLINE_SURFACE ( (
 ( 1.000000000000000000, 0.9238795325112867385, 1.000000000000000000, 0.9238795325112867385, 1.000000000000000000, 0.9238795325112867385, 1.000000000000000000, 0.9238795325112867385, 1.000000000000000000, 0.9238795325112867385, 1.000000000000000000, 0.9238795325112867385, 1.000000000000000000, 0.9238795325112867385, 1.000000000000000000, 0.9238795325112867385, 1.000000000000000000, 0.9238795325112867385, 1.000000000000000000, 0.9238795325112867385, 1.000000000000000000, 0.9238795325112867385, 1.000000000000000000, 0.9238795325112867385, 1.000000000000000000, 0.9238795325112867385, 1.000000000000000000, 0.9238795325112867385, 1.000000000000000000, 0.9238795325112867385, 1.000000000000000000, 0.9238795325112867385, 1.000000000000000000, 0.9238795325112867385, 1.000000000000000000, 0.9238795325112867385, 1.000000000000000000, 0.9238795325112867385, 1.000000000000000000, 0.9238795325112867385, 1.000000000000000000, 0.9238795325112867385, 1.000000000000000000, 0.9238795325112867385, 1.000000000000000000, 0.9238795325112867385, 1.000000000000000000, 0.9238795325112867385, 1.000000000000000000, 0.9238795325112867385, 1.000000000000000000, 0.9238795325112867385, 1.000000000000000000, 0.9238795325112867385, 1.000000000000000000, 0.9238795325112867385, 1.000000000000000000, 0.9238795325112867385, 1.000000000000000000, 0.9238795325112867385, 1.000000000000000000, 0.9238795325112867385, 1.000000000000000000, 0.9238795325112867385, 1.000000000000000000, 0.9238795325112867385, 1.000000000000000000, 0.9238795325112867385, 1.000000000000000000, 0.9238795325112867385, 1.000000000000000000, 0.9238795325112867385, 1.000000000000000000, 0.9238795325112867385, 1.000000000000000000, 0.9238795325112867385, 1.000000000000000000, 0.9238795325112867385, 1.000000000000000000, 0.9238795325112867385, 1.000000000000000000),
 ( 1.000000000000000000, 0.9238795325112867385, 1.000000000000000000, 0.9238795325112867385, 1.000000000000000000, 0.9238795325112867385, 1.000000000000000000, 0.9238795325112867385, 1.000000000000000000, 0.9238795325112867385, 1.000000000000000000, 0.9238795325112867385, 1.000000000000000000, 0.9238795325112867385, 1.000000000000000000, 0.9238795325112867385, 1.000000000000000000, 0.9238795325112867385, 1.000000000000000000, 0.9238795325112867385, 1.000000000000000000, 0.9238795325112867385, 1.000000000000000000, 0.9238795325112867385, 1.000000000000000000, 0.9238795325112867385, 1.000000000000000000, 0.9238795325112867385, 1.000000000000000000, 0.9238795325112867385, 1.000000000000000000, 0.9238795325112867385, 1.000000000000000000, 0.9238795325112867385, 1.000000000000000000, 0.9238795325112867385, 1.000000000000000000, 0.9238795325112867385, 1.000000000000000000, 0.9238795325112867385, 1.000000000000000000, 0.9238795325112867385, 1.000000000000000000, 0.9238795325112867385, 1.000000000000000000, 0.9238795325112867385, 1.000000000000000000, 0.9238795325112867385, 1.000000000000000000, 0.9238795325112867385, 1.000000000000000000, 0.9238795325112867385, 1.000000000000000000, 0.9238795325112867385, 1.000000000000000000, 0.9238795325112867385, 1.000000000000000000, 0.9238795325112867385, 1.000000000000000000, 0.9238795325112867385, 1.000000000000000000, 0.9238795325112867385, 1.000000000000000000, 0.9238795325112867385, 1.000000000000000000, 0.9238795325112867385, 1.000000000000000000, 0.9238795325112867385, 1.000000000000000000, 0.9238795325112867385, 1.000000000000000000, 0.9238795325112867385, 1.000000000000000000, 0.9238795325112867385, 1.000000000000000000, 0.9238795325112867385, 1.000000000000000000, 0.9238795325112867385, 1.000000000000000000, 0.9238795325112867385, 1.000000000000000000) ) ) 
 REPRESENTATION_ITEM ( '' )  SURFACE ( )  );
#8222=CARTESIAN_POINT ( 'NONE',  ( -25.00000000000000000, 5.049999998088170017, -10.35533905932738108 ) ) ;
#8224=( GEOMETRIC_REPRESENTATION_CONTEXT ( 3 ) GLOBAL_UNCERTAINTY_ASSIGNED_CONTEXT ( ( #5715 ) ) GLOBAL_UNIT_ASSIGNED_CONTEXT ( ( #1890, #9565, #6098 ) ) REPRESENTATION_CONTEXT ( 'NONE', 'WORKASPACE' ) );
#8243=CARTESIAN_POINT ( 'NONE',  ( -17.40975659021753330, 1.843749999044084653, 17.40975659021752975 ) ) ;
#8254=DIRECTION ( 'NONE',  ( 0.000000000000000000, 0.000000000000000000, -1.000000000000000000 ) ) ;
#8260=CARTESIAN_POINT ( 'NONE',  ( -10.19839929293505776, 0.7062499990440845865, -24.62111388750000174 ) ) ;
#8265=CARTESIAN_POINT ( 'NONE',  ( 17.67766952966369232, 2.737499998088169573, -17.67766952966369232 ) ) ;
#8275=CARTESIAN_POINT ( 'NONE',  ( -25.00000000000000000, 4.049999998088169129, -10.35533905932738108 ) ) ;
#8276=CARTESIAN_POINT ( 'NONE',  ( 24.62111388749999463, 5.156249999044083765, 10.19839929293507730 ) ) ;
#8278=ORIENTED_EDGE ( 'NONE', *, *, #1096, .F. ) ;
#8290=ORIENTED_EDGE ( 'NONE', *, *, #10707, .F. ) ;
#8297=ORIENTED_EDGE ( 'NONE', *, *, #9964, .T. ) ;
#8301=CARTESIAN_POINT ( 'NONE',  ( 17.40975659021752620, 3.093749999044084653, 17.40975659021753330 ) ) ;
#8313=CARTESIAN_POINT ( 'NONE',  ( 9.644816411522782573, 5.000000000000000000, 22.72594373997417705 ) ) ;
#8324=CARTESIAN_POINT ( 'NONE',  ( 10.35533905932737930, 3.799999998088170461, -25.00000000000000000 ) ) ;
#8330=AXIS2_PLACEMENT_3D ( 'NONE', #3313, #4064, #6658 ) ;
#8337=CARTESIAN_POINT ( 'NONE',  ( 1.530808498934191521E-15, 3.862499998088169573, -25.00000000000000000 ) ) ;
#8341=ORIENTED_EDGE ( 'NONE', *, *, #10388, .T. ) ;
#8347=CIRCLE ( 'NONE', #3588, 22.00000000000000355 ) ;
#8353=ORIENTED_EDGE ( 'NONE', *, *, #7467, .T. ) ;
#8356=UNCERTAINTY_MEASURE_WITH_UNIT (LENGTH_MEASURE( 1.000000000000000082E-05 ), #6637, 'distance_accuracy_value', 'NONE');
#8360=CARTESIAN_POINT ( 'NONE',  ( 0.000000000000000000, -58.00000000000000000, -24.91176187412963117 ) ) ;
#8362=DIRECTION ( 'NONE',  ( 0.000000000000000000, -1.000000000000000000, 0.000000000000000000 ) ) ;
#8363=CARTESIAN_POINT ( 'NONE',  ( 17.40975659021752975, 2.343749999044085097, -17.40975659021752975 ) ) ;
#8402=CARTESIAN_POINT ( 'NONE',  ( 10.19839929293505953, 0.4062499990440845421, -24.62111388750000174 ) ) ;
#8407=EDGE_CURVE ( 'NONE', #292, #9493, #1252, .T. ) ;
#8411=CARTESIAN_POINT ( 'NONE',  ( -17.40975659021753330, 3.843749999044085097, 17.40975659021752975 ) ) ;
#8429=CARTESIAN_POINT ( 'NONE',  ( -19.05903902044739695, 4.999999999999999112, -16.17878337876688022 ) ) ;
#8430=CARTESIAN_POINT ( 'NONE',  ( -10.35533905932741128, 4.312500000000000888, -24.99999999999996803 ) ) ;
#8439=CARTESIAN_POINT ( 'NONE',  ( -24.62111388750000174, 1.831249999044084475, -10.19839929293506131 ) ) ;
#8445=DIRECTION ( 'NONE',  ( 0.000000000000000000, -1.000000000000000000, 0.000000000000000000 ) ) ;
#8457=CARTESIAN_POINT ( 'NONE',  ( 17.40975659021752620, 2.268749999044084475, 17.40975659021753330 ) ) ;
#8463=DIRECTION ( 'NONE',  ( 0.000000000000000000, 0.000000000000000000, -1.000000000000000000 ) ) ;
#8466=CARTESIAN_POINT ( 'NONE',  ( 17.67766952966369232, 0.1249999999999999722, -17.67766952966369232 ) ) ;
#8472=( GEOMETRIC_REPRESENTATION_CONTEXT ( 3 ) GLOBAL_UNCERTAINTY_ASSIGNED_CONTEXT ( ( #70 ) ) GLOBAL_UNIT_ASSIGNED_CONTEXT ( ( #3920, #2243, #1420 ) ) REPRESENTATION_CONTEXT ( 'NONE', 'WORKASPACE' ) );
#8474=ADVANCED_FACE ( 'NONE', ( #8195 ), #627, .T. ) ;
#8483=CARTESIAN_POINT ( 'NONE',  ( 24.62111388750000174, 0.3937499990440845310, 0.000000000000000000 ) ) ;
#8490=FACE_OUTER_BOUND ( 'NONE', #1244, .T. ) ;
#8492=EDGE_CURVE ( 'NONE', #9493, #10743, #10072, .T. ) ;
#8498=CARTESIAN_POINT ( 'NONE',  ( 17.40975659021752975, 1.518749999044084698, -17.40975659021752975 ) ) ;
#8504=SHAPE_REPRESENTATION_RELATIONSHIP ( 'NONE' , 'NONE' ,  #4232, #5075 ) ;
#8506=CARTESIAN_POINT ( 'NONE',  ( -10.35533905932737575, 1.924999998088169129, -25.00000000000000000 ) ) ;
#8508=CARTESIAN_POINT ( 'NONE',  ( 25.00000000000000000, 4.000000000000000000, 0.000000000000000000 ) ) ;
#8516=CARTESIAN_POINT ( 'NONE',  ( 10.19839929293506486, 4.206249999044085364, 24.62111388749999819 ) ) ;
#8528=CARTESIAN_POINT ( 'NONE',  ( 25.00000000000000000, 1.000000000000000000, 0.000000000000000000 ) ) ;
#8539=CYLINDRICAL_SURFACE ( 'NONE', #2014, 25.00000000000000000 ) ;
#8542=CARTESIAN_POINT ( 'NONE',  ( 22.35845142874864422, 5.000000000000000000, 10.92382174880114754 ) ) ;
#8548=CARTESIAN_POINT ( 'NONE',  ( 1.507608415688466075E-15, 2.643749999044084920, -24.62111388750000174 ) ) ;
#8549=ORIENTED_EDGE ( 'NONE', *, *, #3463, .F. ) ;
#8556=CARTESIAN_POINT ( 'NONE',  ( 10.19839929293505953, 2.581249999044084475, -24.62111388750000174 ) ) ;
#8560=EDGE_LOOP ( 'NONE', ( #487, #8152, #1583, #7358 ) ) ;
#8565=CARTESIAN_POINT ( 'NONE',  ( -25.00000000000001421, 1.174999998088169351, 10.35533905932737397 ) ) ;
#8567=CARTESIAN_POINT ( 'NONE',  ( -25.00000000000000000, 3.500000000000000000, -3.061616997868383043E-15 ) ) ;
#8572=CARTESIAN_POINT ( 'NONE',  ( 17.40975659021752620, 4.268749999044085364, 17.40975659021753330 ) ) ;
#8581=FACE_OUTER_BOUND ( 'NONE', #834, .T. ) ;
#8582=CARTESIAN_POINT ( 'NONE',  ( -17.67766952966368876, 1.375000000000000000, -17.67766952966369232 ) ) ;
#8586=ORIENTED_EDGE ( 'NONE', *, *, #7007, .T. ) ;
#8588=( BOUNDED_CURVE ( )  B_SPLINE_CURVE ( 2, ( #3592, #1120, #10338, #166, #889, #9326, #10215, #9266, #5090 ),
 .UNSPECIFIED., .F., .F. ) 
 B_SPLINE_CURVE_WITH_KNOTS ( ( 3, 2, 2, 2, 3 ),
 ( 0.05000000000000000278, 0.07499999999999999722, 0.1000000000000000056, 0.1250000000000000000, 0.1499999999999999944 ),
 .UNSPECIFIED. ) 
 CURVE ( )  GEOMETRIC_REPRESENTATION_ITEM ( )  RATIONAL_B_SPLINE_CURVE ( ( 1.000000000000000000, 0.9238795325112867385, 1.000000000000000000, 0.9238795325112867385, 1.000000000000000000, 0.9238795325112867385, 1.000000000000000000, 0.9238795325112867385, 1.000000000000000000 ) ) 
 REPRESENTATION_ITEM ( '' )  );
#8601=EDGE_CURVE ( 'NONE', #2611, #2038, #5913, .T. ) ;
#8604=CARTESIAN_POINT ( 'NONE',  ( -24.62111388750000174, 3.893749999044084475, -3.015216831376932151E-15 ) ) ;
#8614=CARTESIAN_POINT ( 'NONE',  ( 1.507608415688466075E-15, 1.643749999044084475, -24.62111388750000174 ) ) ;
#8615=CARTESIAN_POINT ( 'NONE',  ( 24.62111388750000174, 1.393749999044084475, 0.000000000000000000 ) ) ;
#8624=CARTESIAN_POINT ( 'NONE',  ( 25.00000000000000000, 3.000000000000000000, 0.000000000000000000 ) ) ;
#8629=CARTESIAN_POINT ( 'NONE',  ( -10.19839929293505776, 4.706249999044086252, -24.62111388750000174 ) ) ;
#8635=ORIENTED_EDGE ( 'NONE', *, *, #2925, .F. ) ;
#8641=CARTESIAN_POINT ( 'NONE',  ( -24.62111388750000884, 4.781249999044083765, 10.19839929293505421 ) ) ;
#8648=CARTESIAN_POINT ( 'NONE',  ( 0.000000000000000000, 5.000000000000000000, -25.00000000000000000 ) ) ;
#8649=VECTOR ( 'NONE', #2134, 1000.000000000000000 ) ;
#8656=CARTESIAN_POINT ( 'NONE',  ( 0.000000000000000000, -55.00000000000000000, 24.91176187412963117 ) ) ;
#8667=CARTESIAN_POINT ( 'NONE',  ( -17.40975659021753330, 1.018749999044084698, 17.40975659021752975 ) ) ;
#8677=DIRECTION ( 'NONE',  ( 0.000000000000000000, -1.000000000000000000, 0.000000000000000000 ) ) ;
#8680=DIRECTION ( 'NONE',  ( 0.000000000000000000, -1.000000000000000000, 0.000000000000000000 ) ) ;
#8681=CARTESIAN_POINT ( 'NONE',  ( 24.62111388750000174, 0.2187499990440845699, 0.000000000000000000 ) ) ;
#8682=CARTESIAN_POINT ( 'NONE',  ( -4.592425496802574367E-15, 1.362499998088169129, 25.00000000000000000 ) ) ;
#8684=EDGE_CURVE ( 'NONE', #3847, #2572, #5160, .T. ) ;
#8691=CARTESIAN_POINT ( 'NONE',  ( 1.507608415688466075E-15, 1.468749999044084431, -24.62111388750000174 ) ) ;
#8701=CARTESIAN_POINT ( 'NONE',  ( -4.592425496802574367E-15, 1.750000000000000000, 25.00000000000000000 ) ) ;
#8702=ADVANCED_FACE ( 'NONE', ( #1907 ), #6944, .F. ) ;
#8712=AXIS2_PLACEMENT_3D ( 'NONE', #6299, #1172, #5373 ) ;
#8726=CARTESIAN_POINT ( 'NONE',  ( 24.99999999999999289, 1.549999998088169129, 10.35533905932739529 ) ) ;
#8727=CARTESIAN_POINT ( 'NONE',  ( -17.40975659021753330, 3.018749999044084475, 17.40975659021752975 ) ) ;
#8733=ORIENTED_EDGE ( 'NONE', *, *, #10707, .T. ) ;
#8734=EDGE_CURVE ( 'NONE', #1424, #10065, #5624, .T. ) ;
#8737=CARTESIAN_POINT ( 'NONE',  ( -24.26769393075472436, 4.999999999999999112, 5.061130139468667188 ) ) ;
#8742=CARTESIAN_POINT ( 'NONE',  ( 17.40975659021752975, 4.343749999044084653, -17.40975659021752975 ) ) ;
#8743=DIRECTION ( 'NONE',  ( 0.000000000000000000, 0.000000000000000000, -1.000000000000000000 ) ) ;
#8747=CARTESIAN_POINT ( 'NONE',  ( -10.19839929293505776, 2.531249999044085097, -24.62111388750000174 ) ) ;
#8754=FACE_OUTER_BOUND ( 'NONE', #7582, .T. ) ;
#8763=CARTESIAN_POINT ( 'NONE',  ( 1.530808498934191521E-15, 3.862499998088169573, -25.00000000000000000 ) ) ;
#8766=DIRECTION ( 'NONE',  ( 0.000000000000000000, -1.000000000000000000, 0.000000000000000000 ) ) ;
#8772=ORIENTED_EDGE ( 'NONE', *, *, #8067, .T. ) ;
#8773=CARTESIAN_POINT ( 'NONE',  ( -17.40975659021753330, 4.018749999044084475, 17.40975659021752975 ) ) ;
#8780=VECTOR ( 'NONE', #8863, 999.9999999999998863 ) ;
#8790=CARTESIAN_POINT ( 'NONE',  ( -17.40975659021752975, 4.593749999044084653, -17.40975659021752975 ) ) ;
#8795=VECTOR ( 'NONE', #6357, 1000.000000000000000 ) ;
#8796=CARTESIAN_POINT ( 'NONE',  ( 10.19839929293505953, 3.406249999044085097, -24.62111388750000174 ) ) ;
#8827=CARTESIAN_POINT ( 'NONE',  ( -4.592425496802574367E-15, 1.750000000000000000, 25.00000000000000000 ) ) ;
#8833=CARTESIAN_POINT ( 'NONE',  ( 24.62111388750000174, 5.393749999044085364, 0.000000000000000000 ) ) ;
#8841=CARTESIAN_POINT ( 'NONE',  ( 10.19839929293506486, 3.031249999044084653, 24.62111388749999819 ) ) ;
#8847=CARTESIAN_POINT ( 'NONE',  ( -24.62111388750000174, 4.718749999044084653, -3.015216831376932151E-15 ) ) ;
#8849=VERTEX_POINT ( 'NONE', #3831 ) ;
#8855=CARTESIAN_POINT ( 'NONE',  ( 3.418204983771597728E-15, -8.000000000000000000, 27.91176187412962761 ) ) ;
#8857=CARTESIAN_POINT ( 'NONE',  ( -25.00000000000000000, 2.500000000000000000, -3.061616997868383043E-15 ) ) ;
#8863=DIRECTION ( 'NONE',  ( 0.000000000000000000, -0.9396926207859082059, -0.3420201433256694901 ) ) ;
#8876=DIRECTION ( 'NONE',  ( 0.000000000000000000, -1.000000000000000000, 0.000000000000000000 ) ) ;
#8880=VECTOR ( 'NONE', #434, 1000.000000000000000 ) ;
#8886=ORIENTED_EDGE ( 'NONE', *, *, #4926, .F. ) ;
#8896=CARTESIAN_POINT ( 'NONE',  ( 24.62111388750000174, 3.218749999044084653, 0.000000000000000000 ) ) ;
#8898=EDGE_CURVE ( 'NONE', #6538, #2980, #5168, .T. ) ;
#8900=ORIENTED_EDGE ( 'NONE', *, *, #8601, .T. ) ;
#8903=CARTESIAN_POINT ( 'NONE',  ( -10.19839929293505776, 4.531249999044084653, -24.62111388750000174 ) ) ;
#8924=VERTEX_POINT ( 'NONE', #8855 ) ;
#8925=CARTESIAN_POINT ( 'NONE',  ( -19.05903902044739695, 4.999999999999999112, -16.17878337876688022 ) ) ;
#8926=CARTESIAN_POINT ( 'NONE',  ( 25.00000000000000000, 0.6124999980881691286, 0.000000000000000000 ) ) ;
#8928=CARTESIAN_POINT ( 'NONE',  ( 3.061616997868383043E-15, 5.000000000000000000, 25.00000000000000000 ) ) ;
#8933=( BOUNDED_CURVE ( )  B_SPLINE_CURVE ( 2, ( #4307, #98, #9097, #1528, #3224, #8260, #704, #4083, #10824, #6621, #8667, #9379, #1051, #1821, #7902, #10380, #9443, #1169, #1876, #7851, #2685, #5255, #6190, #10433, #2740, #2793, #3637, #5207, #9555, #6085, #10328, #7021, #6249, #3518, #6973, #1992, #8548, #1214, #10488, #5368, #7124, #5310, #8727, #325, #9609, #4546, #6133, #2041, #4595, #3692, #275, #7074, #3580, #2848, #1110, #9498, #8604, #5415, #8773, #995, #4491, #7945, #376, #3745, #6022, #1932, #218, #4360, #7725, #4423, #7788, #158, #6914, #10267, #480 ),
 .UNSPECIFIED., .F., .F. ) 
 B_SPLINE_CURVE_WITH_KNOTS ( ( 3, 2, 2, 2, 2, 2, 2, 2, 2, 2, 2, 2, 2, 2, 2, 2, 2, 2, 2, 2, 2, 2, 2, 2, 2, 2, 2, 2, 2, 2, 2, 2, 2, 2, 2, 2, 2, 3 ),
 ( 0.000000000000000000, 0.02500000000000000139, 0.05000000000000000278, 0.07499999999999999722, 0.1000000000000000056, 0.1250000000000000000, 0.1499999999999999944, 0.1749999999999999889, 0.2000000000000000111, 0.2250000000000000056, 0.2500000000000000000, 0.2750000000000000222, 0.2999999999999999889, 0.3250000000000000111, 0.3499999999999999778, 0.3750000000000000000, 0.4000000000000000222, 0.4249999999999999889, 0.4500000000000000111, 0.4749999999999999778, 0.5000000000000000000, 0.5250000000000000222, 0.5500000000000000444, 0.5749999999999999556, 0.5999999999999999778, 0.6250000000000000000, 0.6500000000000000222, 0.6750000000000000444, 0.6999999999999999556, 0.7249999999999999778, 0.7500000000000000000, 0.7750000000000000222, 0.8000000000000000444, 0.8249999999999999556, 0.8499999999999999778, 0.8750000000000000000, 0.9000000000000000222, 0.9210736448048598701 ),
 .UNSPECIFIED. ) 
 CURVE ( )  GEOMETRIC_REPRESENTATION_ITEM ( )  RATIONAL_B_SPLINE_CURVE ( ( 1.000000000000000000, 0.9238795325112867385, 1.000000000000000000, 0.9238795325112867385, 1.000000000000000000, 0.9238795325112867385, 1.000000000000000000, 0.9238795325112867385, 1.000000000000000000, 0.9238795325112867385, 1.000000000000000000, 0.9238795325112867385, 1.000000000000000000, 0.9238795325112867385, 1.000000000000000000, 0.9238795325112867385, 1.000000000000000000, 0.9238795325112867385, 1.000000000000000000, 0.9238795325112867385, 1.000000000000000000, 0.9238795325112867385, 1.000000000000000000, 0.9238795325112867385, 1.000000000000000000, 0.9238795325112867385, 1.000000000000000000, 0.9238795325112867385, 1.000000000000000000, 0.9238795325112867385, 1.000000000000000000, 0.9238795325112867385, 1.000000000000000000, 0.9238795325112867385, 1.000000000000000000, 0.9238795325112867385, 1.000000000000000000, 0.9238795325112867385, 1.000000000000000000, 0.9238795325112867385, 1.000000000000000000, 0.9238795325112867385, 1.000000000000000000, 0.9238795325112867385, 1.000000000000000000, 0.9238795325112867385, 1.000000000000000000, 0.9238795325112867385, 1.000000000000000000, 0.9238795325112867385, 1.000000000000000000, 0.9238795325112867385, 1.000000000000000000, 0.9238795325112867385, 1.000000000000000000, 0.9238795325112867385, 1.000000000000000000, 0.9238795325112867385, 1.000000000000000000, 0.9238795325112867385, 1.000000000000000000, 0.9238795325112867385, 1.000000000000000000, 0.9238795325112867385, 1.000000000000000000, 0.9238795325112867385, 1.000000000000000000, 0.9238795325112867385, 1.000000000000000000, 0.9238795325112867385, 1.000000000000000000, 0.9238795325112867385, 1.000000000000000000, 0.9358345722305186909, 0.9798450991463130144 ) ) 
 REPRESENTATION_ITEM ( '' )  );
#8943=CARTESIAN_POINT ( 'NONE',  ( 10.19839929293505953, 3.406249999044085097, -24.62111388750000174 ) ) ;
#8951=CARTESIAN_POINT ( 'NONE',  ( -4.522825247065398226E-15, 1.143749999044084475, 24.62111388750000174 ) ) ;
#8971=AXIS2_PLACEMENT_3D ( 'NONE', #1579, #763, #7497 ) ;
#8993=CARTESIAN_POINT ( 'NONE',  ( 1.530808498934191521E-15, 3.862499998088169573, -25.00000000000000000 ) ) ;
#8995=CARTESIAN_POINT ( 'NONE',  ( 10.35533905932738286, 2.424999998088169129, 24.99999999999999645 ) ) ;
#9004=CARTESIAN_POINT ( 'NONE',  ( 17.67766952966369232, 4.737499998088169129, -17.67766952966369232 ) ) ;
#9018=ORIENTED_EDGE ( 'NONE', *, *, #2585, .T. ) ;
#9023=CARTESIAN_POINT ( 'NONE',  ( 24.62111388750000174, 0.2187499990440845699, 0.000000000000000000 ) ) ;
#9024=ORIENTED_EDGE ( 'NONE', *, *, #1723, .F. ) ;
#9028=CARTESIAN_POINT ( 'NONE',  ( 17.40975659021752620, 4.093749999044084653, 17.40975659021753330 ) ) ;
#9029=CARTESIAN_POINT ( 'NONE',  ( -17.67766952966368876, 3.375000000000000000, -17.67766952966369232 ) ) ;
#9037=CIRCLE ( 'NONE', #739, 22.00000000000000355 ) ;
#9041=CYLINDRICAL_SURFACE ( 'NONE', #2022, 24.91176187412963117 ) ;
#9044=CARTESIAN_POINT ( 'NONE',  ( 24.81055694375000087, 0.1093749995220422710, 0.000000000000000000 ) ) ;
#9046=AXIS2_PLACEMENT_3D ( 'NONE', #7308, #10688, #4062 ) ;
#9049=ORIENTED_EDGE ( 'NONE', *, *, #4926, .T. ) ;
#9050=AXIS2_PLACEMENT_3D ( 'NONE', #9691, #8088, #3238 ) ;
#9057=DIRECTION ( 'NONE',  ( 0.000000000000000000, -1.000000000000000000, 0.000000000000000000 ) ) ;
#9064=CARTESIAN_POINT ( 'NONE',  ( 25.00000000000000000, 3.612499998088169129, 0.000000000000000000 ) ) ;
#9072=ORIENTED_EDGE ( 'NONE', *, *, #7389, .F. ) ;
#9076=CARTESIAN_POINT ( 'NONE',  ( 17.67766952966369232, 3.125000000000000000, -17.67766952966369232 ) ) ;
#9081=CARTESIAN_POINT ( 'NONE',  ( 24.62111388749999463, 3.156249999044084653, 10.19839929293507730 ) ) ;
#9088=CYLINDRICAL_SURFACE ( 'NONE', #5203, 25.00000000000000000 ) ;
#9091=CARTESIAN_POINT ( 'NONE',  ( 10.35533905932739174, 0.8125000000000001110, 24.99999999999998934 ) ) ;
#9097=CARTESIAN_POINT ( 'NONE',  ( 17.40975659021752975, 0.5187499990440845865, -17.40975659021752975 ) ) ;
#9101=CARTESIAN_POINT ( 'NONE',  ( 17.67766952966368521, 2.487499998088169129, 17.67766952966369232 ) ) ;
#9106=ORIENTED_EDGE ( 'NONE', *, *, #5552, .T. ) ;
#9108=CARTESIAN_POINT ( 'NONE',  ( 10.19839929293506486, 5.031249999044083765, 24.62111388749999819 ) ) ;
#9128=CARTESIAN_POINT ( 'NONE',  ( 10.19839929293506486, 1.031249999044084653, 24.62111388749999819 ) ) ;
#9131=CARTESIAN_POINT ( 'NONE',  ( 1.507608415688466075E-15, 1.468749999044084431, -24.62111388750000174 ) ) ;
#9133=EDGE_LOOP ( 'NONE', ( #596, #8549, #4469, #10310, #2000, #9977, #3622, #6643, #8290, #5331, #6608, #9912, #9923 ) ) ;
#9141=DIRECTION ( 'NONE',  ( 0.000000000000000000, 0.000000000000000000, -1.000000000000000000 ) ) ;
#9144=CARTESIAN_POINT ( 'NONE',  ( 1.530808498934191521E-15, 1.862499998088169129, -25.00000000000000000 ) ) ;
#9146=CARTESIAN_POINT ( 'NONE',  ( 12.19759864389371629, 5.000000000000001776, 21.50133847031806411 ) ) ;
#9162=VECTOR ( 'NONE', #7403, 1000.000000000000000 ) ;
#9163=CARTESIAN_POINT ( 'NONE',  ( -10.35533905932737575, 4.924999998088169129, -25.00000000000000000 ) ) ;
#9173=AXIS2_PLACEMENT_3D ( 'NONE', #8147, #7117, #10482 ) ;
#9182=CARTESIAN_POINT ( 'NONE',  ( -10.35533905932736687, 1.924999998088168907, -25.00000000000000711 ) ) ;
#9185=CARTESIAN_POINT ( 'NONE',  ( 17.40975659021752975, 1.343749999044084653, -17.40975659021752975 ) ) ;
#9189=AXIS2_PLACEMENT_3D ( 'NONE', #79, #7480, #2391 ) ;
#9193=CARTESIAN_POINT ( 'NONE',  ( 25.00000000000000000, 5.000000000000000000, 0.000000000000000000 ) ) ;
#9195=CARTESIAN_POINT ( 'NONE',  ( 15.18771902014174735, 5.000000000000000888, 19.59342933435411993 ) ) ;
#9202=CARTESIAN_POINT ( 'NONE',  ( -4.592425496802574367E-15, 1.362499998088169129, 25.00000000000000000 ) ) ;
#9207=CARTESIAN_POINT ( 'NONE',  ( -25.00000000000000000, 1.437500000000000000, -10.35533905932738108 ) ) ;
#9213=ORIENTED_EDGE ( 'NONE', *, *, #7935, .F. ) ;
#9216=CARTESIAN_POINT ( 'NONE',  ( 1.507608415688466075E-15, 4.643749999044084475, -24.62111388750000174 ) ) ;
#9228=AXIS2_PLACEMENT_3D ( 'NONE', #2449, #6614, #8254 ) ;
#9230=VERTEX_POINT ( 'NONE', #8827 ) ;
#9238=CARTESIAN_POINT ( 'NONE',  ( 17.67766952966368521, 4.487499998088169129, 17.67766952966369232 ) ) ;
#9239=CARTESIAN_POINT ( 'NONE',  ( -24.62111388750000174, 3.656249999044084653, -10.19839929293506131 ) ) ;
#9242=ORIENTED_EDGE ( 'NONE', *, *, #5768, .T. ) ;
#9253=CARTESIAN_POINT ( 'NONE',  ( -25.00000000000001066, 4.562500000000001776, 10.35533905932737397 ) ) ;
#9257=CARTESIAN_POINT ( 'NONE',  ( 0.000000000000000000, -58.00000000000000000, 0.000000000000000000 ) ) ;
#9264=CARTESIAN_POINT ( 'NONE',  ( 24.62111388750000174, 2.456249999044084475, -10.19839929293505776 ) ) ;
#9266=CARTESIAN_POINT ( 'NONE',  ( -10.35533905932739174, 1.299999998088168907, 24.99999999999999289 ) ) ;
#9276=EDGE_CURVE ( 'NONE', #10743, #2139, #7432, .T. ) ;
#9281=DIRECTION ( 'NONE',  ( 0.000000000000000000, -0.9396926207859082059, -0.3420201433256694901 ) ) ;
#9282=CARTESIAN_POINT ( 'NONE',  ( 17.40975659021752620, 5.268749999044085364, 17.40975659021753330 ) ) ;
#9290=CARTESIAN_POINT ( 'NONE',  ( 1.530808498934191521E-15, 1.250000000000000000, -25.00000000000000000 ) ) ;
#9302=ORIENTED_EDGE ( 'NONE', *, *, #10388, .F. ) ;
#9303=CARTESIAN_POINT ( 'NONE',  ( 17.67766952966369232, 2.125000000000000000, -17.67766952966369232 ) ) ;
#9305=CARTESIAN_POINT ( 'NONE',  ( -4.592425496802574367E-15, 3.750000000000000000, 25.00000000000000000 ) ) ;
#9307=CARTESIAN_POINT ( 'NONE',  ( 22.95776900584396074, 5.000000000000000000, 9.642149850605726158 ) ) ;
#9313=CARTESIAN_POINT ( 'NONE',  ( -17.67766952966368876, 4.375000000000000000, -17.67766952966369232 ) ) ;
#9315=PLANE ( 'NONE',  #3525 ) ;
#9321=CARTESIAN_POINT ( 'NONE',  ( 10.19839929293506486, 4.206249999044084475, 24.62111388749999819 ) ) ;
#9326=CARTESIAN_POINT ( 'NONE',  ( -25.00000000000001066, 1.174999998088169351, 10.35533905932737397 ) ) ;
#9329=CARTESIAN_POINT ( 'NONE',  ( 10.35533905932737930, 1.799999998088168907, -25.00000000000000000 ) ) ;
#9341=CARTESIAN_POINT ( 'NONE',  ( -4.522825247065398226E-15, 3.143749999044084475, 24.62111388750000174 ) ) ;
#9354=CARTESIAN_POINT ( 'NONE',  ( -10.19839929293505776, 4.531249999044084653, -24.62111388750000174 ) ) ;
#9361=MECHANICAL_DESIGN_GEOMETRIC_PRESENTATION_REPRESENTATION('',(#540),#8472);
#9365=CARTESIAN_POINT ( 'NONE',  ( -25.00000000000000000, 4.112499998088169129, -3.061616997868383043E-15 ) ) ;
#9371=CARTESIAN_POINT ( 'NONE',  ( 24.95478587032620865, 5.000000000000001776, 1.418225997825871554 ) ) ;
#9375=ORIENTED_EDGE ( 'NONE', *, *, #2795, .F. ) ;
#9379=CARTESIAN_POINT ( 'NONE',  ( -10.19839929293507375, 1.081249999044084475, 24.62111388749999108 ) ) ;
#9388=CARTESIAN_POINT ( 'NONE',  ( 17.40975659021752975, 1.518749999044084698, -17.40975659021752975 ) ) ;
#9389=CARTESIAN_POINT ( 'NONE',  ( 17.40975659021752975, 3.518749999044084920, -17.40975659021752975 ) ) ;
#9398=CARTESIAN_POINT ( 'NONE',  ( 25.00000000000000000, 2.612499998088169129, 0.000000000000000000 ) ) ;
#9400=CARTESIAN_POINT ( 'NONE',  ( -17.67766952966368876, 4.375000000000000000, -17.67766952966369232 ) ) ;
#9405=CARTESIAN_POINT ( 'NONE',  ( -10.19839929293505776, 2.706249999044084475, -24.62111388750000174 ) ) ;
#9429=ORIENTED_EDGE ( 'NONE', *, *, #6294, .T. ) ;
#9443=CARTESIAN_POINT ( 'NONE',  ( 24.62111388750000174, 1.393749999044084475, 0.000000000000000000 ) ) ;
#9445=DIRECTION ( 'NONE',  ( 0.000000000000000000, -1.000000000000000000, 0.000000000000000000 ) ) ;
#9447=DIRECTION ( 'NONE',  ( 0.000000000000000000, -1.000000000000000000, 0.000000000000000000 ) ) ;
#9452=CARTESIAN_POINT ( 'NONE',  ( -10.19839929293507552, 2.081249999044084475, 24.62111388749999463 ) ) ;
#9460=CARTESIAN_POINT ( 'NONE',  ( -10.19839929293505776, 0.5312499990440845421, -24.62111388750000174 ) ) ;
#9462=CARTESIAN_POINT ( 'NONE',  ( -10.35533905932739174, 3.687500000000000444, 24.99999999999999289 ) ) ;
#9468=CARTESIAN_POINT ( 'NONE',  ( -24.62111388750000174, 2.893749999044084475, -3.015216831376932151E-15 ) ) ;
#9478=ORIENTED_EDGE ( 'NONE', *, *, #5325, .T. ) ;
#9480=ORIENTED_EDGE ( 'NONE', *, *, #2523, .T. ) ;
#9493=VERTEX_POINT ( 'NONE', #8483 ) ;
#9495=CARTESIAN_POINT ( 'NONE',  ( 10.35533905932738286, 2.812500000000000000, 24.99999999999999645 ) ) ;
#9498=CARTESIAN_POINT ( 'NONE',  ( -24.62111388750000174, 3.831249999044084920, -10.19839929293506131 ) ) ;
#9502=LINE ( 'NONE', #9658, #2885 ) ;
#9508=CARTESIAN_POINT ( 'NONE',  ( 17.40975659021752620, 5.268749999044085364, 17.40975659021753330 ) ) ;
#9513=ORIENTED_EDGE ( 'NONE', *, *, #10521, .F. ) ;
#9519=EDGE_CURVE ( 'NONE', #5115, #2663, #4351, .T. ) ;
#9522=CARTESIAN_POINT ( 'NONE',  ( -4.522825247065398226E-15, 2.143749999044084920, 24.62111388750000174 ) ) ;
#9525=CARTESIAN_POINT ( 'NONE',  ( 24.62111388750000174, 0.2187499990440845699, 0.000000000000000000 ) ) ;
#9532=DIRECTION ( 'NONE',  ( 0.000000000000000000, 0.000000000000000000, -1.000000000000000000 ) ) ;
#9534=CARTESIAN_POINT ( 'NONE',  ( -25.00000000000001421, 1.562500000000000000, 10.35533905932737397 ) ) ;
#9555=CARTESIAN_POINT ( 'NONE',  ( -4.522825247065398226E-15, 2.143749999044084920, 24.62111388750000174 ) ) ;
#9565=( NAMED_UNIT ( * ) PLANE_ANGLE_UNIT ( ) SI_UNIT ( $, .RADIAN. ) );
#9568=CARTESIAN_POINT ( 'NONE',  ( -10.19839929293505776, 1.531249999044084653, -24.62111388750000174 ) ) ;
#9578=CARTESIAN_POINT ( 'NONE',  ( 17.40975659021752975, 4.343749999044084653, -17.40975659021752975 ) ) ;
#9587=CARTESIAN_POINT ( 'NONE',  ( -4.592425496802574367E-15, 2.750000000000000000, 25.00000000000000000 ) ) ;
#9606=AXIS2_PLACEMENT_3D ( 'NONE', #1572, #3326, #10083 ) ;
#9609=CARTESIAN_POINT ( 'NONE',  ( -4.522825247065398226E-15, 3.143749999044084475, 24.62111388750000174 ) ) ;
#9616=CARTESIAN_POINT ( 'NONE',  ( -17.40975659021752975, 4.768749999044084475, -17.40975659021752975 ) ) ;
#9619=DIRECTION ( 'NONE',  ( 0.000000000000000000, -1.000000000000000000, 0.000000000000000000 ) ) ;
#9620=EDGE_LOOP ( 'NONE', ( #4972, #10246, #5420, #5031 ) ) ;
#9623=CARTESIAN_POINT ( 'NONE',  ( -24.62111388750000884, 2.781249999044085097, 10.19839929293505421 ) ) ;
#9625=CARTESIAN_POINT ( 'NONE',  ( 17.67766952966369232, 4.125000000000000000, -17.67766952966369232 ) ) ;
#9630=CARTESIAN_POINT ( 'NONE',  ( -17.40975659021753330, 2.843749999044085097, 17.40975659021752975 ) ) ;
#9640=CARTESIAN_POINT ( 'NONE',  ( 17.67766952966368521, 1.875000000000000000, 17.67766952966369232 ) ) ;
#9648=DIRECTION ( 'NONE',  ( 0.000000000000000000, -1.000000000000000000, 0.000000000000000000 ) ) ;
#9656=( BOUNDED_CURVE ( )  B_SPLINE_CURVE ( 2, ( #8926, #5569, #4018, #9858, #3969 ),
 .UNSPECIFIED., .F., .F. ) 
 B_SPLINE_CURVE_WITH_KNOTS ( ( 3, 2, 3 ),
 ( 0.000000000000000000, 0.02500000000000000486, 0.05000000000000000971 ),
 .UNSPECIFIED. ) 
 CURVE ( )  GEOMETRIC_REPRESENTATION_ITEM ( )  RATIONAL_B_SPLINE_CURVE ( ( 1.000000000000000000, 0.9238795325112867385, 1.000000000000000000, 0.9238795325112867385, 1.000000000000000000 ) ) 
 REPRESENTATION_ITEM ( '' )  );
#9658=CARTESIAN_POINT ( 'NONE',  ( 0.000000000000000000, 5.000000000000000000, -25.00000000000000000 ) ) ;
#9666=AXIS2_PLACEMENT_3D ( 'NONE', #2803, #2144, #7181 ) ;
#9667=CARTESIAN_POINT ( 'NONE',  ( -23.00215391598666059, 5.000000000000000000, 9.113568881329346283 ) ) ;
#9672=CARTESIAN_POINT ( 'NONE',  ( 0.000000000000000000, -58.00000000000000000, 0.000000000000000000 ) ) ;
#9675=CARTESIAN_POINT ( 'NONE',  ( 10.19839929293505953, 1.406249999044084209, -24.62111388750000174 ) ) ;
#9682=CARTESIAN_POINT ( 'NONE',  ( -10.19839929293505776, 1.531249999044084653, -24.62111388750000174 ) ) ;
#9691=CARTESIAN_POINT ( 'NONE',  ( 0.000000000000000000, -55.00000000000000000, 0.000000000000000000 ) ) ;
#9694=EDGE_CURVE ( 'NONE', #8014, #9966, #3844, .T. ) ;
#9716=( BOUNDED_SURFACE ( )  B_SPLINE_SURFACE ( 1, 2, ( 
 ( #5923, #6865, #6986, #6151, #3419, #1951, #4512, #1778, #6101, #8565, #5328, #290, #8682, #6810, #7866, #2581, #5979, #1716, #5096, #9329, #5157, #8506, #7687, #960, #116, #3476, #2704, #10224, #3536, #2641, #4382, #6037, #9398, #7745, #4927, #9940, #3081, #5746, #6474, #1494, #7294, #552, #8180, #9828, #10612, #4823, #4766, #3181, #9064, #10833, #3936, #1542, #8337, #718, #6524, #8275, #5646, #6429, #9779, #3028, #4097, #6580, #10775, #8121, #4875, #2211, #9004, #10670, #1430, #9163, #2262, #8222, #609, #2417, #10716, #7342, #7454, #3232, #1597, #2371, #3990 ),
 ( #3130, #9880, #5591, #6631, #2315, #9989, #779, #1381, #5699, #662, #5800, #4983, #8951, #4149, #4042, #7396, #8615, #5149, #8498, #951, #10213, #52, #1003, #8439, #6029, #1706, #887, #9452, #4198, #4317, #4256, #10944, #4371, #9264, #3349, #8556, #3411, #6803, #3466, #3527, #6746, #7677, #6921, #10161, #107, #6857, #6692, #2632, #2524, #2574, #9389, #10279, #830, #5970, #1832, #5858, #5915, #5213, #6092, #1060, #1884, #9321, #7509, #10887, #3289, #10049, #1772, #2470, #9216, #1659, #9616, #7959, #1174, #3759, #3702, #10443, #2904, #282, #9508, #7136, #8833 ) ),
 .UNSPECIFIED., .F., .F., .F. ) 
 B_SPLINE_SURFACE_WITH_KNOTS ( ( 2, 2 ),
 ( 3, 2, 2, 2, 2, 2, 2, 2, 2, 2, 2, 2, 2, 2, 2, 2, 2, 2, 2, 2, 2, 2, 2, 2, 2, 2, 2, 2, 2, 2, 2, 2, 2, 2, 2, 2, 2, 2, 2, 2, 3 ),
 ( 0.000000000000000000, 1.000000000000000000 ),
 ( 0.000000000000000000, 0.02500000000000000139, 0.05000000000000000278, 0.07499999999999999722, 0.1000000000000000056, 0.1250000000000000000, 0.1499999999999999944, 0.1749999999999999889, 0.2000000000000000111, 0.2250000000000000056, 0.2500000000000000000, 0.2750000000000000222, 0.2999999999999999889, 0.3250000000000000111, 0.3499999999999999778, 0.3750000000000000000, 0.4000000000000000222, 0.4249999999999999889, 0.4500000000000000111, 0.4749999999999999778, 0.5000000000000000000, 0.5250000000000000222, 0.5500000000000000444, 0.5749999999999999556, 0.5999999999999999778, 0.6250000000000000000, 0.6500000000000000222, 0.6750000000000000444, 0.6999999999999999556, 0.7249999999999999778, 0.7500000000000000000, 0.7750000000000000222, 0.8000000000000000444, 0.8249999999999999556, 0.8499999999999999778, 0.8750000000000000000, 0.9000000000000000222, 0.9250000000000000444, 0.9499999999999999556, 0.9749999999999999778, 1.000000000000000000 ),
 .UNSPECIFIED. ) 
 GEOMETRIC_REPRESENTATION_ITEM ( )  RATIONAL_B_SPLINE_SURFACE ( (
 ( 1.000000000000000000, 0.9238795325112867385, 1.000000000000000000, 0.9238795325112867385, 1.000000000000000000, 0.9238795325112867385, 1.000000000000000000, 0.9238795325112867385, 1.000000000000000000, 0.9238795325112867385, 1.000000000000000000, 0.9238795325112867385, 1.000000000000000000, 0.9238795325112867385, 1.000000000000000000, 0.9238795325112867385, 1.000000000000000000, 0.9238795325112867385, 1.000000000000000000, 0.9238795325112867385, 1.000000000000000000, 0.9238795325112867385, 1.000000000000000000, 0.9238795325112867385, 1.000000000000000000, 0.9238795325112867385, 1.000000000000000000, 0.9238795325112867385, 1.000000000000000000, 0.9238795325112867385, 1.000000000000000000, 0.9238795325112867385, 1.000000000000000000, 0.9238795325112867385, 1.000000000000000000, 0.9238795325112867385, 1.000000000000000000, 0.9238795325112867385, 1.000000000000000000, 0.9238795325112867385, 1.000000000000000000, 0.9238795325112867385, 1.000000000000000000, 0.9238795325112867385, 1.000000000000000000, 0.9238795325112867385, 1.000000000000000000, 0.9238795325112867385, 1.000000000000000000, 0.9238795325112867385, 1.000000000000000000, 0.9238795325112867385, 1.000000000000000000, 0.9238795325112867385, 1.000000000000000000, 0.9238795325112867385, 1.000000000000000000, 0.9238795325112867385, 1.000000000000000000, 0.9238795325112867385, 1.000000000000000000, 0.9238795325112867385, 1.000000000000000000, 0.9238795325112867385, 1.000000000000000000, 0.9238795325112867385, 1.000000000000000000, 0.9238795325112867385, 1.000000000000000000, 0.9238795325112867385, 1.000000000000000000, 0.9238795325112867385, 1.000000000000000000, 0.9238795325112867385, 1.000000000000000000, 0.9238795325112867385, 1.000000000000000000, 0.9238795325112867385, 1.000000000000000000, 0.9238795325112867385, 1.000000000000000000),
 ( 1.000000000000000000, 0.9238795325112867385, 1.000000000000000000, 0.9238795325112867385, 1.000000000000000000, 0.9238795325112867385, 1.000000000000000000, 0.9238795325112867385, 1.000000000000000000, 0.9238795325112867385, 1.000000000000000000, 0.9238795325112867385, 1.000000000000000000, 0.9238795325112867385, 1.000000000000000000, 0.9238795325112867385, 1.000000000000000000, 0.9238795325112867385, 1.000000000000000000, 0.9238795325112867385, 1.000000000000000000, 0.9238795325112867385, 1.000000000000000000, 0.9238795325112867385, 1.000000000000000000, 0.9238795325112867385, 1.000000000000000000, 0.9238795325112867385, 1.000000000000000000, 0.9238795325112867385, 1.000000000000000000, 0.9238795325112867385, 1.000000000000000000, 0.9238795325112867385, 1.000000000000000000, 0.9238795325112867385, 1.000000000000000000, 0.9238795325112867385, 1.000000000000000000, 0.9238795325112867385, 1.000000000000000000, 0.9238795325112867385, 1.000000000000000000, 0.9238795325112867385, 1.000000000000000000, 0.9238795325112867385, 1.000000000000000000, 0.9238795325112867385, 1.000000000000000000, 0.9238795325112867385, 1.000000000000000000, 0.9238795325112867385, 1.000000000000000000, 0.9238795325112867385, 1.000000000000000000, 0.9238795325112867385, 1.000000000000000000, 0.9238795325112867385, 1.000000000000000000, 0.9238795325112867385, 1.000000000000000000, 0.9238795325112867385, 1.000000000000000000, 0.9238795325112867385, 1.000000000000000000, 0.9238795325112867385, 1.000000000000000000, 0.9238795325112867385, 1.000000000000000000, 0.9238795325112867385, 1.000000000000000000, 0.9238795325112867385, 1.000000000000000000, 0.9238795325112867385, 1.000000000000000000, 0.9238795325112867385, 1.000000000000000000, 0.9238795325112867385, 1.000000000000000000, 0.9238795325112867385, 1.000000000000000000) ) ) 
 REPRESENTATION_ITEM ( '' )  SURFACE ( )  );
#9718=CARTESIAN_POINT ( 'NONE',  ( -19.96339341614531193, 5.000000000000000888, -15.08987035441359303 ) ) ;
#9725=CARTESIAN_POINT ( 'NONE',  ( 17.40975659021752975, 2.343749999044085097, -17.40975659021752975 ) ) ;
#9728=AXIS2_PLACEMENT_3D ( 'NONE', #2767, #1027, #193 ) ;
#9730=CARTESIAN_POINT ( 'NONE',  ( -17.40975659021752975, 1.593749999044084431, -17.40975659021752975 ) ) ;
#9740=ORIENTED_EDGE ( 'NONE', *, *, #5768, .F. ) ;
#9744=CARTESIAN_POINT ( 'NONE',  ( 0.000000000000000000, 5.000000000000000000, -22.00000000000000355 ) ) ;
#9754=VERTEX_POINT ( 'NONE', #2341 ) ;
#9772=CARTESIAN_POINT ( 'NONE',  ( -10.19839929293507375, 2.906249999044085541, 24.62111388749999108 ) ) ;
#9773=CARTESIAN_POINT ( 'NONE',  ( 25.00000000000000000, -2.710505431213761085E-17, 0.000000000000000000 ) ) ;
#9776=ADVANCED_FACE ( 'NONE', ( #4850 ), #6494, .T. ) ;
#9779=CARTESIAN_POINT ( 'NONE',  ( -17.67766952966369232, 4.237499998088169129, 17.67766952966368876 ) ) ;
#9789=EDGE_CURVE ( 'NONE', #5382, #5890, #7896, .T. ) ;
#9793=CARTESIAN_POINT ( 'NONE',  ( -10.35533905932738108, 0.6875000000000002220, 24.99999999999999645 ) ) ;
#9804=FACE_OUTER_BOUND ( 'NONE', #10788, .T. ) ;
#9815=EDGE_LOOP ( 'NONE', ( #2433, #8772, #7550, #1946 ) ) ;
#9817=PRODUCT_CONTEXT ( 'NONE', #5756, 'mechanical' ) ;
#9828=CARTESIAN_POINT ( 'NONE',  ( -10.35533905932739174, 3.299999998088169129, 24.99999999999999289 ) ) ;
#9850=CARTESIAN_POINT ( 'NONE',  ( -24.62111388750000174, 2.656249999044085097, -10.19839929293506131 ) ) ;
#9858=CARTESIAN_POINT ( 'NONE',  ( 10.35533905932737930, 0.7999999980881692396, -25.00000000000000000 ) ) ;
#9873=CARTESIAN_POINT ( 'NONE',  ( -25.00000000000000000, 1.500000000000000000, -3.061616997868383043E-15 ) ) ;
#9875=ADVANCED_FACE ( 'NONE', ( #16 ), #10135, .T. ) ;
#9880=CARTESIAN_POINT ( 'NONE',  ( 24.62111388750000174, 0.4562499990440845310, -10.19839929293505776 ) ) ;
#9904=DIRECTION ( 'NONE',  ( 0.000000000000000000, -1.000000000000000000, 0.000000000000000000 ) ) ;
#9912=ORIENTED_EDGE ( 'NONE', *, *, #8407, .T. ) ;
#9923=ORIENTED_EDGE ( 'NONE', *, *, #6520, .T. ) ;
#9925=SURFACE_STYLE_FILL_AREA ( #6564 ) ;
#9940=CARTESIAN_POINT ( 'NONE',  ( 10.35533905932737930, 2.799999998088169573, -25.00000000000000000 ) ) ;
#9953=ADVANCED_FACE ( 'NONE', ( #6606 ), #10913, .T. ) ;
#9962=CARTESIAN_POINT ( 'NONE',  ( -10.19839929293507552, 0.9062499990440844311, 24.62111388749999463 ) ) ;
#9964=EDGE_CURVE ( 'NONE', #57, #9754, #10139, .T. ) ;
#9966=VERTEX_POINT ( 'NONE', #1090 ) ;
#9967=VERTEX_POINT ( 'NONE', #2719 ) ;
#9972=CARTESIAN_POINT ( 'NONE',  ( -4.592425496802574367E-15, 0.7500000000000000000, 25.00000000000000000 ) ) ;
#9973=DIRECTION ( 'NONE',  ( 0.000000000000000000, -1.000000000000000000, 0.000000000000000000 ) ) ;
#9975=CARTESIAN_POINT ( 'NONE',  ( 18.31891771041502537, 4.999999999999998224, 16.72517935659742960 ) ) ;
#9977=ORIENTED_EDGE ( 'NONE', *, *, #9964, .F. ) ;
#9984=CYLINDRICAL_SURFACE ( 'NONE', #7469, 27.91176187412963117 ) ;
#9989=CARTESIAN_POINT ( 'NONE',  ( -10.19839929293505776, 0.7062499990440844755, -24.62111388750000174 ) ) ;
#9995=( NAMED_UNIT ( * ) PLANE_ANGLE_UNIT ( ) SI_UNIT ( $, .RADIAN. ) );
#10015=CARTESIAN_POINT ( 'NONE',  ( 10.35533905932734733, 4.799999998088170905, -25.00000000000004263 ) ) ;
#10016=AXIS2_PLACEMENT_3D ( 'NONE', #2477, #3135, #5706 ) ;
#10017=CARTESIAN_POINT ( 'NONE',  ( -24.62111388750000174, 0.7187499990440845421, -3.015216831376932151E-15 ) ) ;
#10049=CARTESIAN_POINT ( 'NONE',  ( 24.62111388750000174, 4.456249999044084475, -10.19839929293505776 ) ) ;
#10060=AXIS2_PLACEMENT_3D ( 'NONE', #3528, #2575, #2696 ) ;
#10065=VERTEX_POINT ( 'NONE', #7764 ) ;
#10067=( BOUNDED_SURFACE ( )  B_SPLINE_SURFACE ( 1, 2, ( 
 ( #2035, #5411, #1355, #1509, #6657, #1462, #3098, #4122, #10017, #743, #5823, #9962, #10690, #6715, #4063, #1624, #2441, #10739, #9185, #3152, #9131, #4008, #8196, #4891, #6547, #7311, #8243, #4849, #10859, #5765, #7531, #629, #5012, #5064, #8363, #3206, #804, #2340, #6493, #9850, #2287, #4170, #3257, #7481, #5722, #10073, #8301, #9081, #686, #10912, #7421, #3312, #5887, #7362, #2488, #9239, #1683, #2392, #8411, #853, #1564, #5668, #9028, #6605, #10802, #5292, #1030, #4404, #1796, #9354, #5177, #2770, #7646, #8641, #10187, #1089, #5997, #10134, #4464, #15, #7763 ),
 ( #6777, #2546, #8466, #2718, #2659, #5939, #6170, #135, #7824, #3555, #80, #10308, #3436, #5238, #4282, #5111, #8528, #2602, #4220, #3498, #9290, #195, #8582, #254, #6947, #9534, #1973, #5343, #8701, #1736, #9640, #6228, #358, #7980, #2170, #4683, #10569, #7157, #1151, #2115, #8857, #4726, #1894, #6039, #10291, #3599, #118, #5274, #8624, #6932, #4384, #1070, #2707, #7747, #6987, #6103, #8567, #175, #4445, #9462, #5159, #1842, #5224, #1015, #8508, #2643, #962, #4327, #7689, #3478, #9400, #6867, #10226, #303, #7928, #7880, #1149, #2658, #6884, #7762, #1908 ) ),
 .UNSPECIFIED., .F., .F., .F. ) 
 B_SPLINE_SURFACE_WITH_KNOTS ( ( 2, 2 ),
 ( 3, 2, 2, 2, 2, 2, 2, 2, 2, 2, 2, 2, 2, 2, 2, 2, 2, 2, 2, 2, 2, 2, 2, 2, 2, 2, 2, 2, 2, 2, 2, 2, 2, 2, 2, 2, 2, 2, 2, 2, 3 ),
 ( 0.000000000000000000, 1.000000000000000000 ),
 ( 0.000000000000000000, 0.02500000000000000139, 0.05000000000000000278, 0.07499999999999999722, 0.1000000000000000056, 0.1250000000000000000, 0.1499999999999999944, 0.1749999999999999889, 0.2000000000000000111, 0.2250000000000000056, 0.2500000000000000000, 0.2750000000000000222, 0.2999999999999999889, 0.3250000000000000111, 0.3499999999999999778, 0.3750000000000000000, 0.4000000000000000222, 0.4249999999999999889, 0.4500000000000000111, 0.4749999999999999778, 0.5000000000000000000, 0.5250000000000000222, 0.5500000000000000444, 0.5749999999999999556, 0.5999999999999999778, 0.6250000000000000000, 0.6500000000000000222, 0.6750000000000000444, 0.6999999999999999556, 0.7249999999999999778, 0.7500000000000000000, 0.7750000000000000222, 0.8000000000000000444, 0.8249999999999999556, 0.8499999999999999778, 0.8750000000000000000, 0.9000000000000000222, 0.9250000000000000444, 0.9499999999999999556, 0.9749999999999999778, 1.000000000000000000 ),
 .UNSPECIFIED. ) 
 GEOMETRIC_REPRESENTATION_ITEM ( )  RATIONAL_B_SPLINE_SURFACE ( (
 ( 1.000000000000000000, 0.9238795325112867385, 1.000000000000000000, 0.9238795325112867385, 1.000000000000000000, 0.9238795325112867385, 1.000000000000000000, 0.9238795325112867385, 1.000000000000000000, 0.9238795325112867385, 1.000000000000000000, 0.9238795325112867385, 1.000000000000000000, 0.9238795325112867385, 1.000000000000000000, 0.9238795325112867385, 1.000000000000000000, 0.9238795325112867385, 1.000000000000000000, 0.9238795325112867385, 1.000000000000000000, 0.9238795325112867385, 1.000000000000000000, 0.9238795325112867385, 1.000000000000000000, 0.9238795325112867385, 1.000000000000000000, 0.9238795325112867385, 1.000000000000000000, 0.9238795325112867385, 1.000000000000000000, 0.9238795325112867385, 1.000000000000000000, 0.9238795325112867385, 1.000000000000000000, 0.9238795325112867385, 1.000000000000000000, 0.9238795325112867385, 1.000000000000000000, 0.9238795325112867385, 1.000000000000000000, 0.9238795325112867385, 1.000000000000000000, 0.9238795325112867385, 1.000000000000000000, 0.9238795325112867385, 1.000000000000000000, 0.9238795325112867385, 1.000000000000000000, 0.9238795325112867385, 1.000000000000000000, 0.9238795325112867385, 1.000000000000000000, 0.9238795325112867385, 1.000000000000000000, 0.9238795325112867385, 1.000000000000000000, 0.9238795325112867385, 1.000000000000000000, 0.9238795325112867385, 1.000000000000000000, 0.9238795325112867385, 1.000000000000000000, 0.9238795325112867385, 1.000000000000000000, 0.9238795325112867385, 1.000000000000000000, 0.9238795325112867385, 1.000000000000000000, 0.9238795325112867385, 1.000000000000000000, 0.9238795325112867385, 1.000000000000000000, 0.9238795325112867385, 1.000000000000000000, 0.9238795325112867385, 1.000000000000000000, 0.9238795325112867385, 1.000000000000000000, 0.9238795325112867385, 1.000000000000000000),
 ( 1.000000000000000000, 0.9238795325112867385, 1.000000000000000000, 0.9238795325112867385, 1.000000000000000000, 0.9238795325112867385, 1.000000000000000000, 0.9238795325112867385, 1.000000000000000000, 0.9238795325112867385, 1.000000000000000000, 0.9238795325112867385, 1.000000000000000000, 0.9238795325112867385, 1.000000000000000000, 0.9238795325112867385, 1.000000000000000000, 0.9238795325112867385, 1.000000000000000000, 0.9238795325112867385, 1.000000000000000000, 0.9238795325112867385, 1.000000000000000000, 0.9238795325112867385, 1.000000000000000000, 0.9238795325112867385, 1.000000000000000000, 0.9238795325112867385, 1.000000000000000000, 0.9238795325112867385, 1.000000000000000000, 0.9238795325112867385, 1.000000000000000000, 0.9238795325112867385, 1.000000000000000000, 0.9238795325112867385, 1.000000000000000000, 0.9238795325112867385, 1.000000000000000000, 0.9238795325112867385, 1.000000000000000000, 0.9238795325112867385, 1.000000000000000000, 0.9238795325112867385, 1.000000000000000000, 0.9238795325112867385, 1.000000000000000000, 0.9238795325112867385, 1.000000000000000000, 0.9238795325112867385, 1.000000000000000000, 0.9238795325112867385, 1.000000000000000000, 0.9238795325112867385, 1.000000000000000000, 0.9238795325112867385, 1.000000000000000000, 0.9238795325112867385, 1.000000000000000000, 0.9238795325112867385, 1.000000000000000000, 0.9238795325112867385, 1.000000000000000000, 0.9238795325112867385, 1.000000000000000000, 0.9238795325112867385, 1.000000000000000000, 0.9238795325112867385, 1.000000000000000000, 0.9238795325112867385, 1.000000000000000000, 0.9238795325112867385, 1.000000000000000000, 0.9238795325112867385, 1.000000000000000000, 0.9238795325112867385, 1.000000000000000000, 0.9238795325112867385, 1.000000000000000000, 0.9238795325112867385, 1.000000000000000000) ) ) 
 REPRESENTATION_ITEM ( '' )  SURFACE ( )  );
#10071=CARTESIAN_POINT ( 'NONE',  ( -12.67266974794317491, 5.000000000000000888, 21.23116648297597209 ) ) ;
#10072=LINE ( 'NONE', #7584, #7605 ) ;
#10073=CARTESIAN_POINT ( 'NONE',  ( 10.19839929293506486, 3.031249999044084653, 24.62111388749999819 ) ) ;
#10074=CARTESIAN_POINT ( 'NONE',  ( 0.000000000000000000, 5.000000000000000000, 0.000000000000000000 ) ) ;
#10083=DIRECTION ( 'NONE',  ( 0.000000000000000000, 0.000000000000000000, -1.000000000000000000 ) ) ;
#10116=FACE_OUTER_BOUND ( 'NONE', #9133, .T. ) ;
#10127=CARTESIAN_POINT ( 'NONE',  ( -24.62111388750000174, 0.7187499990440845421, -3.015216831376932151E-15 ) ) ;
#10134=CARTESIAN_POINT ( 'NONE',  ( 10.19839929293506486, 5.031249999044083765, 24.62111388749999819 ) ) ;
#10135=CYLINDRICAL_SURFACE ( 'NONE', #8330, 25.00000000000000000 ) ;
#10138=VERTEX_POINT ( 'NONE', #2712 ) ;
#10139=( BOUNDED_CURVE ( )  B_SPLINE_CURVE ( 2, ( #913, #4283, #7647, #5178, #81, #6828, #197, #1974, #1909 ),
 .UNSPECIFIED., .F., .F. ) 
 B_SPLINE_CURVE_WITH_KNOTS ( ( 3, 2, 2, 2, 3 ),
 ( 0.4500000000000000111, 0.4749999999999999778, 0.5000000000000000000, 0.5250000000000000222, 0.5500000000000000444 ),
 .UNSPECIFIED. ) 
 CURVE ( )  GEOMETRIC_REPRESENTATION_ITEM ( )  RATIONAL_B_SPLINE_CURVE ( ( 1.000000000000000000, 0.9238795325112867385, 1.000000000000000000, 0.9238795325112867385, 1.000000000000000000, 0.9238795325112867385, 1.000000000000000000, 0.9238795325112867385, 1.000000000000000000 ) ) 
 REPRESENTATION_ITEM ( '' )  );
#10142=CARTESIAN_POINT ( 'NONE',  ( 17.67766952966368521, 1.875000000000000000, 17.67766952966369232 ) ) ;
#10143=CARTESIAN_POINT ( 'NONE',  ( 10.35533905932742016, 4.812499999999999112, 24.99999999999996447 ) ) ;
#10145=CARTESIAN_POINT ( 'NONE',  ( 25.00000000000000000, 5.000000000000000000, 0.000000000000000000 ) ) ;
#10146=PRODUCT_DEFINITION ( 'UNKNOWN', '', #7061, #733 ) ;
#10148=FACE_OUTER_BOUND ( 'NONE', #7250, .T. ) ;
#10152=DIRECTION ( 'NONE',  ( 0.000000000000000000, 0.000000000000000000, -1.000000000000000000 ) ) ;
#10154=DIRECTION ( 'NONE',  ( 0.000000000000000000, 0.000000000000000000, 1.000000000000000000 ) ) ;
#10155=CARTESIAN_POINT ( 'NONE',  ( 25.00000000000000000, 0.3062499990440845643, 0.000000000000000000 ) ) ;
#10159=ORIENTED_EDGE ( 'NONE', *, *, #4743, .F. ) ;
#10160=CARTESIAN_POINT ( 'NONE',  ( 10.19839929293506486, 1.206249999044084698, 24.62111388749999819 ) ) ;
#10161=CARTESIAN_POINT ( 'NONE',  ( -10.19839929293507552, 3.081249999044084475, 24.62111388749999463 ) ) ;
#10176=CARTESIAN_POINT ( 'NONE',  ( -10.19839929293507552, 3.081249999044084475, 24.62111388749999463 ) ) ;
#10187=CARTESIAN_POINT ( 'NONE',  ( -17.40975659021753330, 4.843749999044083765, 17.40975659021752975 ) ) ;
#10196=CARTESIAN_POINT ( 'NONE',  ( 25.00000000000000000, 2.062500000000000000, -10.35533905932737753 ) ) ;
#10200=CARTESIAN_POINT ( 'NONE',  ( 20.96888409245972440, 4.999999999999998224, 13.39592759827673518 ) ) ;
#10209=CARTESIAN_POINT ( 'NONE',  ( 0.000000000000000000, 5.000000000000000000, 0.000000000000000000 ) ) ;
#10213=CARTESIAN_POINT ( 'NONE',  ( 1.507608415688466075E-15, 1.643749999044084475, -24.62111388750000174 ) ) ;
#10215=CARTESIAN_POINT ( 'NONE',  ( -17.67766952966369232, 1.237499998088169129, 17.67766952966368876 ) ) ;
#10220=SURFACE_SIDE_STYLE ('',( #10342 ) ) ;
#10224=CARTESIAN_POINT ( 'NONE',  ( -10.35533905932739174, 2.299999998088168685, 24.99999999999999289 ) ) ;
#10226=CARTESIAN_POINT ( 'NONE',  ( -25.00000000000000000, 4.500000000000000888, -3.061616997868383043E-15 ) ) ;
#10231=ORIENTED_EDGE ( 'NONE', *, *, #7258, .T. ) ;
#10234=CARTESIAN_POINT ( 'NONE',  ( -17.40975659021753330, 0.8437499990440846531, 17.40975659021752975 ) ) ;
#10246=ORIENTED_EDGE ( 'NONE', *, *, #204, .F. ) ;
#10265=CARTESIAN_POINT ( 'NONE',  ( -17.67766952966368876, 4.987499998088170017, -17.67766952966369232 ) ) ;
#10267=CARTESIAN_POINT ( 'NONE',  ( -24.62111388750000884, 4.945761085427167636, 8.486877225504324329 ) ) ;
#10268=DIRECTION ( 'NONE',  ( 0.000000000000000000, -0.000000000000000000, -1.000000000000000000 ) ) ;
#10277=CARTESIAN_POINT ( 'NONE',  ( 17.40975659021752620, 1.268749999044084698, 17.40975659021753330 ) ) ;
#10279=CARTESIAN_POINT ( 'NONE',  ( 10.19839929293505953, 3.581249999044085364, -24.62111388750000174 ) ) ;
#10291=CARTESIAN_POINT ( 'NONE',  ( -4.592425496802574367E-15, 2.750000000000000000, 25.00000000000000000 ) ) ;
#10295=ORIENTED_EDGE ( 'NONE', *, *, #7682, .F. ) ;
#10297=CARTESIAN_POINT ( 'NONE',  ( 1.507608415688466075E-15, 4.643749999044085364, -24.62111388750000174 ) ) ;
#10305=CARTESIAN_POINT ( 'NONE',  ( 24.81055694375000087, 0.1093749995220422710, 0.000000000000000000 ) ) ;
#10308=CARTESIAN_POINT ( 'NONE',  ( -10.35533905932739174, 0.6875000000000000000, 24.99999999999999289 ) ) ;
#10310=ORIENTED_EDGE ( 'NONE', *, *, #7007, .F. ) ;
#10311=ORIENTED_EDGE ( 'NONE', *, *, #5552, .F. ) ;
#10313=EDGE_CURVE ( 'NONE', #1642, #9966, #1062, .T. ) ;
#10317=CARTESIAN_POINT ( 'NONE',  ( 0.000000000000000000, 5.000000000000000000, 0.000000000000000000 ) ) ;
#10318=EDGE_CURVE ( 'NONE', #39, #6463, #8588, .T. ) ;
#10328=CARTESIAN_POINT ( 'NONE',  ( 17.40975659021752620, 2.268749999044084475, 17.40975659021753330 ) ) ;
#10333=CARTESIAN_POINT ( 'NONE',  ( 3.418204983771598122E-15, -58.00000000000000000, -27.91176187412963117 ) ) ;
#10335=CARTESIAN_POINT ( 'NONE',  ( -17.40975659021753330, 1.018749999044084698, 17.40975659021752975 ) ) ;
#10338=CARTESIAN_POINT ( 'NONE',  ( -17.67766952966368876, 0.9874999980881691286, -17.67766952966369232 ) ) ;
#10342=SURFACE_STYLE_FILL_AREA ( #893 ) ;
#10348=CARTESIAN_POINT ( 'NONE',  ( 24.62111388749999463, 5.331249999044085364, 10.19839929293507730 ) ) ;
#10362=STYLED_ITEM ( 'NONE', ( #5219 ), #5075 ) ;
#10374=ORIENTED_EDGE ( 'NONE', *, *, #204, .T. ) ;
#10380=CARTESIAN_POINT ( 'NONE',  ( 24.62111388749999108, 1.331249999044084475, 10.19839929293507730 ) ) ;
#10388=EDGE_CURVE ( 'NONE', #2980, #5115, #7191, .T. ) ;
#10396=CARTESIAN_POINT ( 'NONE',  ( -4.522825247065398226E-15, 0.9687499990440845421, 24.62111388750000174 ) ) ;
#10402=CARTESIAN_POINT ( 'NONE',  ( 17.40975659021752620, 2.093749999044084653, 17.40975659021753330 ) ) ;
#10408=CARTESIAN_POINT ( 'NONE',  ( -25.00000000000000000, 2.500000000000000000, -3.061616997868383043E-15 ) ) ;
#10411=AXIS2_PLACEMENT_3D ( 'NONE', #2929, #3832, #560 ) ;
#10417=AXIS2_PLACEMENT_3D ( 'NONE', #10209, #5140, #10152 ) ;
#10421=DIRECTION ( 'NONE',  ( 0.000000000000000000, 0.000000000000000000, 1.000000000000000000 ) ) ;
#10433=CARTESIAN_POINT ( 'NONE',  ( -24.62111388750000174, 1.831249999044084475, -10.19839929293506131 ) ) ;
#10438=EDGE_CURVE ( 'NONE', #5323, #6538, #10529, .T. ) ;
#10443=CARTESIAN_POINT ( 'NONE',  ( -10.19839929293507552, 5.081249999044084475, 24.62111388749999463 ) ) ;
#10444=DIRECTION ( 'NONE',  ( 0.000000000000000000, 0.000000000000000000, 1.000000000000000000 ) ) ;
#10445=CARTESIAN_POINT ( 'NONE',  ( -24.82160728492508639, 5.000000000000000888, 0.8552643272782575190 ) ) ;
#10450=CARTESIAN_POINT ( 'NONE',  ( 1.507608415688466075E-15, 3.468749999044085097, -24.62111388750000174 ) ) ;
#10451=CARTESIAN_POINT ( 'NONE',  ( 25.00000000000000000, 0.06249999999999997224, -10.35533905932737753 ) ) ;
#10454=ORIENTED_EDGE ( 'NONE', *, *, #7389, .T. ) ;
#10461=CARTESIAN_POINT ( 'NONE',  ( 10.19839929293505953, 2.406249999044085541, -24.62111388750000174 ) ) ;
#10476=DIRECTION ( 'NONE',  ( 4.188538737677001009E-17, -0.9396926207859082059, 0.3420201433256694901 ) ) ;
#10481=CYLINDRICAL_SURFACE ( 'NONE', #1289, 27.91176187412963117 ) ;
#10482=DIRECTION ( 'NONE',  ( 0.000000000000000000, 0.000000000000000000, -1.000000000000000000 ) ) ;
#10488=CARTESIAN_POINT ( 'NONE',  ( -17.40975659021752975, 2.768749999044084475, -17.40975659021752975 ) ) ;
#10501=CARTESIAN_POINT ( 'NONE',  ( 0.000000000000000000, -8.528980942125402365, 0.000000000000000000 ) ) ;
#10503=CARTESIAN_POINT ( 'NONE',  ( -17.40975659021753330, 3.843749999044085097, 17.40975659021752975 ) ) ;
#10514=CARTESIAN_POINT ( 'NONE',  ( -24.62111388750000174, 1.718749999044084431, -3.015216831376932151E-15 ) ) ;
#10521=EDGE_CURVE ( 'NONE', #3614, #10892, #765, .T. ) ;
#10529=B_SPLINE_CURVE_WITH_KNOTS ( 'NONE', 3,
 ( #1275, #338, #6359, #3704, #9667, #4553, #8737, #1224, #10445, #7859, #7961, #2004, #3808, #2093, #8053, #1176, #9718, #1369 ),
 .UNSPECIFIED., .F., .F.,
 ( 4, 2, 2, 2, 2, 2, 2, 2, 4 ),
 ( 0.000000000000000000, 0.004245714814779292905, 0.008491429629558585809, 0.01273714444433788305, 0.01698285925911717509, 0.02122857407389646886, 0.02547428888867576263, 0.02972000370345505293, 0.03396571851823434324 ),
 .UNSPECIFIED. ) ;
#10534=EDGE_LOOP ( 'NONE', ( #1628, #1871, #10586, #676, #10374, #9242, #3672, #7171, #5425, #1393, #7169, #563, #6398, #5403 ) ) ;
#10538=DIRECTION ( 'NONE',  ( 0.000000000000000000, 0.000000000000000000, -1.000000000000000000 ) ) ;
#10553=CARTESIAN_POINT ( 'NONE',  ( -10.19839929293507375, 3.906249999044085097, 24.62111388749999108 ) ) ;
#10559=CYLINDRICAL_SURFACE ( 'NONE', #5318, 24.91176187412963117 ) ;
#10560=CARTESIAN_POINT ( 'NONE',  ( 1.507608415688466075E-15, 3.468749999044085097, -24.62111388750000174 ) ) ;
#10569=CARTESIAN_POINT ( 'NONE',  ( 1.530808498934191521E-15, 2.250000000000000444, -25.00000000000000000 ) ) ;
#10574=CARTESIAN_POINT ( 'NONE',  ( -10.35533905932737575, 0.3125000000000000000, -25.00000000000000000 ) ) ;
#10577=EDGE_CURVE ( 'NONE', #7487, #3376, #3142, .T. ) ;
#10586=ORIENTED_EDGE ( 'NONE', *, *, #9276, .T. ) ;
#10608=CARTESIAN_POINT ( 'NONE',  ( -10.19839929293505776, 2.531249999044085097, -24.62111388750000174 ) ) ;
#10612=CARTESIAN_POINT ( 'NONE',  ( -4.592425496802574367E-15, 3.362499998088169129, 25.00000000000000000 ) ) ;
#10613=CARTESIAN_POINT ( 'NONE',  ( -10.19839929293507552, 4.906249999044083765, 24.62111388749999463 ) ) ;
#10624=ORIENTED_EDGE ( 'NONE', *, *, #3463, .T. ) ;
#10627=CARTESIAN_POINT ( 'NONE',  ( -25.00000000000000000, 0.4374999999999999445, -10.35533905932738108 ) ) ;
#10630=CARTESIAN_POINT ( 'NONE',  ( 1.530808498934191521E-15, 1.862499998088169129, -25.00000000000000000 ) ) ;
#10632=CARTESIAN_POINT ( 'NONE',  ( -4.592425496802574367E-15, 4.362499998088169129, 25.00000000000000000 ) ) ;
#10638=CARTESIAN_POINT ( 'NONE',  ( -10.35533905932739174, 3.687500000000000444, 24.99999999999999289 ) ) ;
#10641=AXIS2_PLACEMENT_3D ( 'NONE', #9672, #5270, #2097 ) ;
#10651=CARTESIAN_POINT ( 'NONE',  ( 17.67766952966369232, 1.125000000000000222, -17.67766952966369232 ) ) ;
#10653=AXIS2_PLACEMENT_3D ( 'NONE', #3217, #9973, #9141 ) ;
#10659=CARTESIAN_POINT ( 'NONE',  ( 0.000000000000000000, 5.000000000000000000, -22.00000000000000355 ) ) ;
#10670=CARTESIAN_POINT ( 'NONE',  ( 10.35533905932737930, 4.799999998088169129, -25.00000000000000000 ) ) ;
#10680=ORIENTED_EDGE ( 'NONE', *, *, #50, .F. ) ;
#10684=CARTESIAN_POINT ( 'NONE',  ( 10.35533905932738286, 3.812500000000000000, 24.99999999999999645 ) ) ;
#10688=DIRECTION ( 'NONE',  ( 0.000000000000000000, -1.000000000000000000, 0.000000000000000000 ) ) ;
#10690=CARTESIAN_POINT ( 'NONE',  ( -4.522825247065398226E-15, 0.9687499990440845421, 24.62111388750000174 ) ) ;
#10701=ORIENTED_EDGE ( 'NONE', *, *, #3989, .T. ) ;
#10707=EDGE_CURVE ( 'NONE', #6463, #5838, #5839, .T. ) ;
#10716=CARTESIAN_POINT ( 'NONE',  ( -17.67766952966369232, 5.237499998088169129, 17.67766952966368876 ) ) ;
#10734=CARTESIAN_POINT ( 'NONE',  ( 10.35533905932737930, 3.187500000000000444, -25.00000000000000000 ) ) ;
#10735=CARTESIAN_POINT ( 'NONE',  ( 10.35533905932738641, 1.799999998088168685, -24.99999999999999289 ) ) ;
#10737=FACE_OUTER_BOUND ( 'NONE', #5567, .T. ) ;
#10739=CARTESIAN_POINT ( 'NONE',  ( 24.62111388750000174, 1.281249999044084653, -10.19839929293505776 ) ) ;
#10743=VERTEX_POINT ( 'NONE', #9023 ) ;
#10766=CARTESIAN_POINT ( 'NONE',  ( -4.592425496802574367E-15, 1.750000000000000000, 25.00000000000000000 ) ) ;
#10775=CARTESIAN_POINT ( 'NONE',  ( 17.67766952966368521, 4.487499998088169129, 17.67766952966369232 ) ) ;
#10788=EDGE_LOOP ( 'NONE', ( #9072, #5346, #2961, #7943 ) ) ;
#10802=CARTESIAN_POINT ( 'NONE',  ( 24.62111388750000174, 4.218749999044084653, 0.000000000000000000 ) ) ;
#10812=CARTESIAN_POINT ( 'NONE',  ( 0.000000000000000000, -0.5289809421253948152, 0.000000000000000000 ) ) ;
#10813=CARTESIAN_POINT ( 'NONE',  ( -4.592425496802574367E-15, 4.750000000000000000, 25.00000000000000000 ) ) ;
#10824=CARTESIAN_POINT ( 'NONE',  ( -24.62111388750000174, 0.8937499990440845865, -3.015216831376932151E-15 ) ) ;
#10833=CARTESIAN_POINT ( 'NONE',  ( 25.00000000000000000, 3.674999998088170017, -10.35533905932737753 ) ) ;
#10850=( BOUNDED_CURVE ( )  B_SPLINE_CURVE ( 2, ( #10909, #9182, #4280, #1620, #5008, #2544, #5109, #3433, #4217 ),
 .UNSPECIFIED., .F., .F. ) 
 B_SPLINE_CURVE_WITH_KNOTS ( ( 3, 2, 2, 2, 3 ),
 ( 0.2499999999999999722, 0.2750000000000000222, 0.2999999999999999889, 0.3250000000000000111, 0.3499999999999999778 ),
 .UNSPECIFIED. ) 
 CURVE ( )  GEOMETRIC_REPRESENTATION_ITEM ( )  RATIONAL_B_SPLINE_CURVE ( ( 1.000000000000000000, 0.9238795325112866275, 1.000000000000000000, 0.9238795325112867385, 1.000000000000000000, 0.9238795325112867385, 1.000000000000000000, 0.9238795325112867385, 1.000000000000000000 ) ) 
 REPRESENTATION_ITEM ( '' )  );
#10859=CARTESIAN_POINT ( 'NONE',  ( -4.522825247065398226E-15, 1.968749999044084653, 24.62111388750000174 ) ) ;
#10861=VERTEX_POINT ( 'NONE', #4945 ) ;
#10868=CARTESIAN_POINT ( 'NONE',  ( 10.19839929293506486, 2.206249999044084920, 24.62111388749999819 ) ) ;
#10873=CARTESIAN_POINT ( 'NONE',  ( 22.03074295656257320, 5.000000000000000000, 11.55328354274170444 ) ) ;
#10875=ORIENTED_EDGE ( 'NONE', *, *, #3248, .T. ) ;
#10887=CARTESIAN_POINT ( 'NONE',  ( 24.62111388749999463, 4.331249999044084475, 10.19839929293507730 ) ) ;
#10892=VERTEX_POINT ( 'NONE', #800 ) ;
#10909=CARTESIAN_POINT ( 'NONE',  ( 1.530808498934191521E-15, 1.862499998088169129, -25.00000000000000000 ) ) ;
#10912=CARTESIAN_POINT ( 'NONE',  ( 24.62111388750000174, 3.281249999044085097, -10.19839929293505776 ) ) ;
#10913=CYLINDRICAL_SURFACE ( 'NONE', #4825, 25.00000000000000000 ) ;
#10917=( BOUNDED_CURVE ( )  B_SPLINE_CURVE ( 2, ( #3386, #924, #10142, #3507, #5947, #10196, #9303, #4294, #7657 ),
 .UNSPECIFIED., .F., .F. ) 
 B_SPLINE_CURVE_WITH_KNOTS ( ( 3, 2, 2, 2, 3 ),
 ( 0.3500000000000000333, 0.3750000000000000555, 0.4000000000000000222, 0.4249999999999999889, 0.4500000000000000111 ),
 .UNSPECIFIED. ) 
 CURVE ( )  GEOMETRIC_REPRESENTATION_ITEM ( )  RATIONAL_B_SPLINE_CURVE ( ( 0.9999999999999997780, 0.9238795325112869605, 1.000000000000000000, 0.9238795325112867385, 1.000000000000000000, 0.9238795325112867385, 1.000000000000000000, 0.9238795325112867385, 1.000000000000000000 ) ) 
 REPRESENTATION_ITEM ( '' )  );
#10927=CARTESIAN_POINT ( 'NONE',  ( 23.22996358440884990, 5.000000000000000000, 8.988974415371478344 ) ) ;
#10944=CARTESIAN_POINT ( 'NONE',  ( 24.62111388749999463, 2.331249999044084031, 10.19839929293507730 ) ) ;
ENDSEC;
END-ISO-10303-21;
